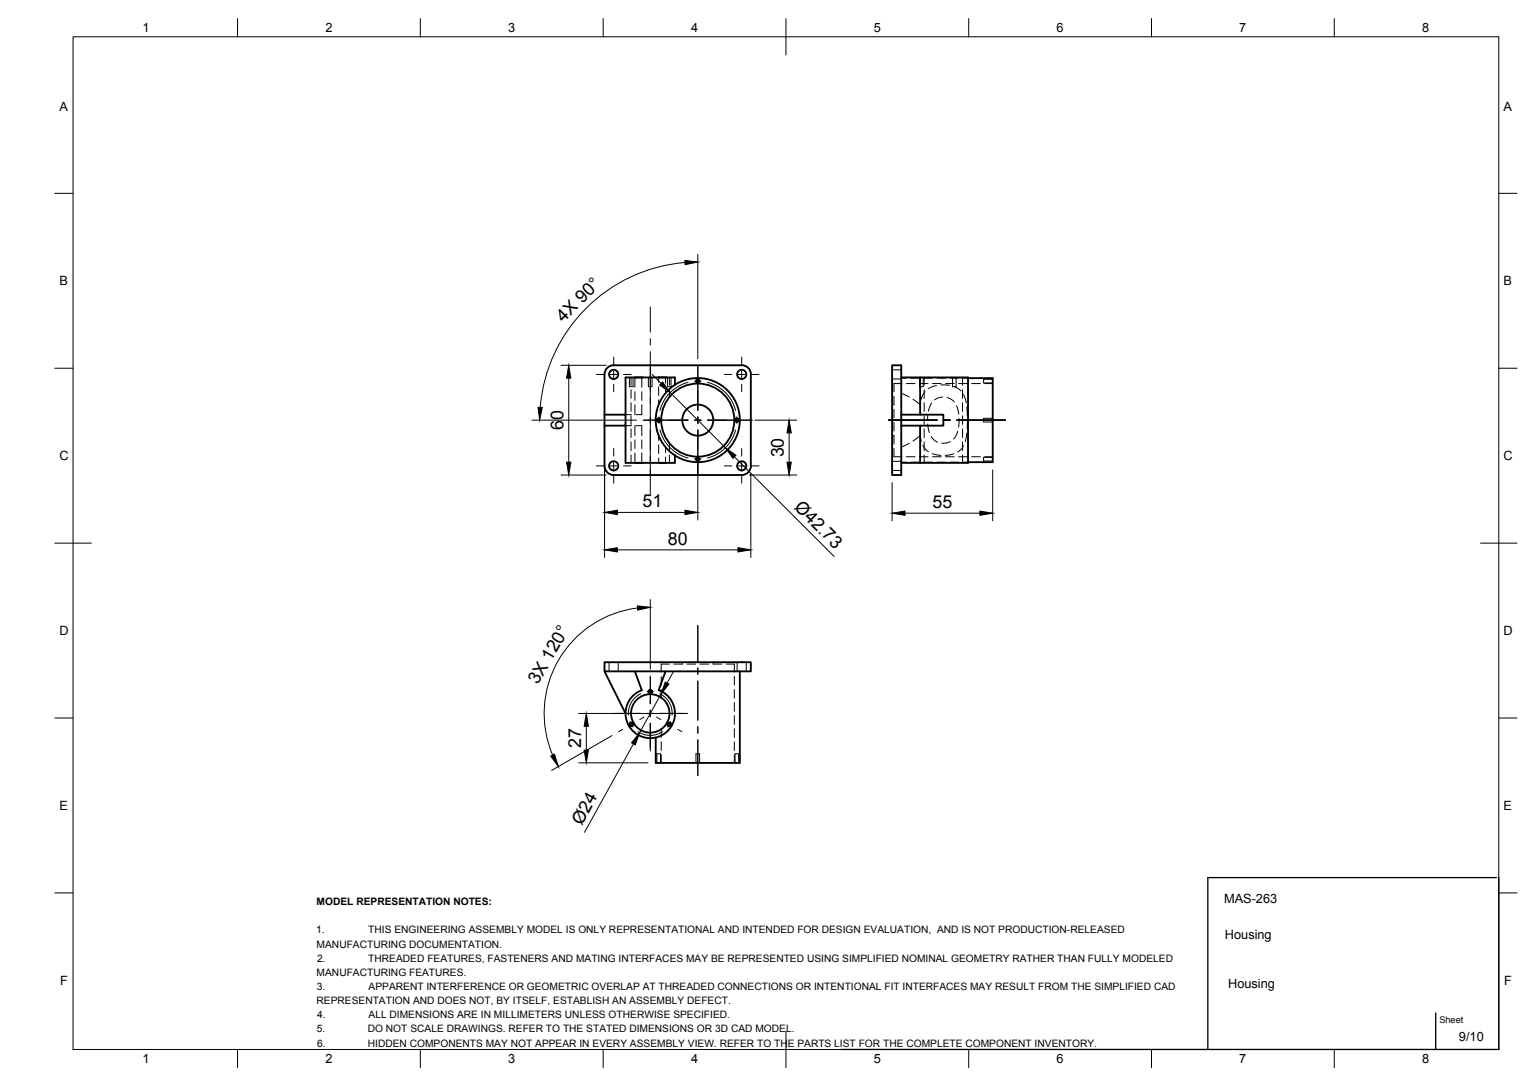
ISO-10303-21;
HEADER;
/* Generated by software containing ST-Developer
 * from STEP Tools, Inc. (www.steptools.com) 
 */

FILE_DESCRIPTION(
/* description */ (''),
/* implementation_level */ '2;1');

FILE_NAME(
/* name */ 'Housing.step',
/* time_stamp */ '2026-10-12T15:47:30-07:00',
/* author */ (''),
/* organization */ (''),
/* preprocessor_version */ 'ST-DEVELOPER v20.2',
/* originating_system */ 'Autodesk Translation Framework v15.15.0.0',
/* authorisation */ '');

FILE_SCHEMA (('AUTOMOTIVE_DESIGN { 1 0 10303 214 3 1 1 }'));
ENDSEC;

DATA;
#10=MECHANICAL_DESIGN_GEOMETRIC_PRESENTATION_REPRESENTATION('',(#87),#88483);
#69=SHAPE_REPRESENTATION_RELATIONSHIP('SRR','None',#88525,#78);
#78=ADVANCED_BREP_SHAPE_REPRESENTATION('',(#122),#88479);
#87=STYLED_ITEM('',(#88574),#122);
#122=MANIFOLD_SOLID_BREP('Body1',#12997);
#240=ELLIPSE('',#13948,67.247501203751,23.);
#241=ELLIPSE('',#13950,67.247501203751,23.);
#378=FACE_BOUND('',#1974,.T.);
#379=FACE_BOUND('',#1975,.T.);
#380=FACE_BOUND('',#1976,.T.);
#381=FACE_BOUND('',#1977,.T.);
#382=FACE_BOUND('',#1995,.T.);
#383=FACE_BOUND('',#1999,.T.);
#384=FACE_BOUND('',#2001,.T.);
#385=FACE_BOUND('',#2003,.T.);
#386=FACE_BOUND('',#2004,.T.);
#387=FACE_BOUND('',#2005,.T.);
#388=FACE_BOUND('',#2006,.T.);
#389=FACE_BOUND('',#2007,.T.);
#390=FACE_BOUND('',#2010,.T.);
#391=FACE_BOUND('',#2011,.T.);
#392=FACE_BOUND('',#2012,.T.);
#393=FACE_BOUND('',#2013,.T.);
#394=FACE_BOUND('',#2015,.T.);
#395=FACE_BOUND('',#2016,.T.);
#396=FACE_BOUND('',#2017,.T.);
#397=FACE_BOUND('',#2018,.T.);
#398=FACE_BOUND('',#2019,.T.);
#525=PLANE('',#13880);
#526=PLANE('',#13884);
#527=PLANE('',#13888);
#528=PLANE('',#13892);
#529=PLANE('',#13899);
#530=PLANE('',#13903);
#531=PLANE('',#13907);
#532=PLANE('',#13923);
#533=PLANE('',#13929);
#534=PLANE('',#13934);
#535=PLANE('',#13937);
#536=PLANE('',#13938);
#537=PLANE('',#13940);
#538=PLANE('',#13941);
#539=PLANE('',#13946);
#540=PLANE('',#13947);
#541=PLANE('',#13949);
#542=PLANE('',#13951);
#543=PLANE('',#13954);
#544=PLANE('',#13955);
#545=PLANE('',#13957);
#546=PLANE('',#13959);
#547=PLANE('',#13962);
#548=PLANE('',#13966);
#549=PLANE('',#13969);
#550=PLANE('',#13970);
#1256=FACE_OUTER_BOUND('',#1953,.T.);
#1257=FACE_OUTER_BOUND('',#1954,.T.);
#1258=FACE_OUTER_BOUND('',#1955,.T.);
#1259=FACE_OUTER_BOUND('',#1956,.T.);
#1260=FACE_OUTER_BOUND('',#1957,.T.);
#1261=FACE_OUTER_BOUND('',#1958,.T.);
#1262=FACE_OUTER_BOUND('',#1959,.T.);
#1263=FACE_OUTER_BOUND('',#1960,.T.);
#1264=FACE_OUTER_BOUND('',#1961,.T.);
#1265=FACE_OUTER_BOUND('',#1962,.T.);
#1266=FACE_OUTER_BOUND('',#1963,.T.);
#1267=FACE_OUTER_BOUND('',#1964,.T.);
#1268=FACE_OUTER_BOUND('',#1965,.T.);
#1269=FACE_OUTER_BOUND('',#1966,.T.);
#1270=FACE_OUTER_BOUND('',#1967,.T.);
#1271=FACE_OUTER_BOUND('',#1968,.T.);
#1272=FACE_OUTER_BOUND('',#1969,.T.);
#1273=FACE_OUTER_BOUND('',#1970,.T.);
#1274=FACE_OUTER_BOUND('',#1971,.T.);
#1275=FACE_OUTER_BOUND('',#1972,.T.);
#1276=FACE_OUTER_BOUND('',#1973,.T.);
#1277=FACE_OUTER_BOUND('',#1978,.T.);
#1278=FACE_OUTER_BOUND('',#1979,.T.);
#1279=FACE_OUTER_BOUND('',#1980,.T.);
#1280=FACE_OUTER_BOUND('',#1981,.T.);
#1281=FACE_OUTER_BOUND('',#1982,.T.);
#1282=FACE_OUTER_BOUND('',#1983,.T.);
#1283=FACE_OUTER_BOUND('',#1984,.T.);
#1284=FACE_OUTER_BOUND('',#1985,.T.);
#1285=FACE_OUTER_BOUND('',#1986,.T.);
#1286=FACE_OUTER_BOUND('',#1987,.T.);
#1287=FACE_OUTER_BOUND('',#1988,.T.);
#1288=FACE_OUTER_BOUND('',#1989,.T.);
#1289=FACE_OUTER_BOUND('',#1990,.T.);
#1290=FACE_OUTER_BOUND('',#1991,.T.);
#1291=FACE_OUTER_BOUND('',#1992,.T.);
#1292=FACE_OUTER_BOUND('',#1993,.T.);
#1293=FACE_OUTER_BOUND('',#1994,.T.);
#1294=FACE_OUTER_BOUND('',#1996,.T.);
#1295=FACE_OUTER_BOUND('',#1997,.T.);
#1296=FACE_OUTER_BOUND('',#1998,.T.);
#1297=FACE_OUTER_BOUND('',#2000,.T.);
#1298=FACE_OUTER_BOUND('',#2002,.T.);
#1299=FACE_OUTER_BOUND('',#2008,.T.);
#1300=FACE_OUTER_BOUND('',#2009,.T.);
#1301=FACE_OUTER_BOUND('',#2014,.T.);
#1953=EDGE_LOOP('',(#11238,#11239,#11240,#11241));
#1954=EDGE_LOOP('',(#11242));
#1955=EDGE_LOOP('',(#11243,#11244,#11245,#11246));
#1956=EDGE_LOOP('',(#11247));
#1957=EDGE_LOOP('',(#11248,#11249,#11250,#11251));
#1958=EDGE_LOOP('',(#11252));
#1959=EDGE_LOOP('',(#11253,#11254,#11255,#11256));
#1960=EDGE_LOOP('',(#11257));
#1961=EDGE_LOOP('',(#11258,#11259,#11260,#11261));
#1962=EDGE_LOOP('',(#11262,#11263,#11264,#11265));
#1963=EDGE_LOOP('',(#11266));
#1964=EDGE_LOOP('',(#11267,#11268,#11269,#11270));
#1965=EDGE_LOOP('',(#11271));
#1966=EDGE_LOOP('',(#11272,#11273,#11274,#11275));
#1967=EDGE_LOOP('',(#11276));
#1968=EDGE_LOOP('',(#11277,#11278,#11279,#11280));
#1969=EDGE_LOOP('',(#11281,#11282,#11283,#11284));
#1970=EDGE_LOOP('',(#11285,#11286,#11287,#11288));
#1971=EDGE_LOOP('',(#11289,#11290,#11291,#11292));
#1972=EDGE_LOOP('',(#11293,#11294,#11295,#11296));
#1973=EDGE_LOOP('',(#11297,#11298,#11299,#11300,#11301,#11302,#11303,#11304,
#11305,#11306,#11307,#11308,#11309,#11310,#11311,#11312,#11313,#11314,#11315));
#1974=EDGE_LOOP('',(#11316));
#1975=EDGE_LOOP('',(#11317));
#1976=EDGE_LOOP('',(#11318));
#1977=EDGE_LOOP('',(#11319));
#1978=EDGE_LOOP('',(#11320,#11321,#11322,#11323));
#1979=EDGE_LOOP('',(#11324,#11325,#11326,#11327));
#1980=EDGE_LOOP('',(#11328,#11329,#11330,#11331));
#1981=EDGE_LOOP('',(#11332,#11333,#11334,#11335,#11336,#11337));
#1982=EDGE_LOOP('',(#11338,#11339,#11340,#11341));
#1983=EDGE_LOOP('',(#11342,#11343,#11344,#11345));
#1984=EDGE_LOOP('',(#11346,#11347,#11348,#11349));
#1985=EDGE_LOOP('',(#11350,#11351,#11352,#11353));
#1986=EDGE_LOOP('',(#11354,#11355,#11356,#11357));
#1987=EDGE_LOOP('',(#11358,#11359,#11360,#11361,#11362,#11363,#11364,#11365,
#11366,#11367));
#1988=EDGE_LOOP('',(#11368,#11369,#11370,#11371));
#1989=EDGE_LOOP('',(#11372,#11373,#11374,#11375));
#1990=EDGE_LOOP('',(#11376,#11377,#11378,#11379));
#1991=EDGE_LOOP('',(#11380,#11381,#11382,#11383,#11384));
#1992=EDGE_LOOP('',(#11385,#11386,#11387,#11388));
#1993=EDGE_LOOP('',(#11389,#11390,#11391,#11392));
#1994=EDGE_LOOP('',(#11393,#11394,#11395));
#1995=EDGE_LOOP('',(#11396));
#1996=EDGE_LOOP('',(#11397,#11398,#11399,#11400));
#1997=EDGE_LOOP('',(#11401,#11402,#11403,#11404,#11405,#11406,#11407,#11408,
#11409));
#1998=EDGE_LOOP('',(#11410));
#1999=EDGE_LOOP('',(#11411));
#2000=EDGE_LOOP('',(#11412,#11413,#11414,#11415));
#2001=EDGE_LOOP('',(#11416,#11417,#11418));
#2002=EDGE_LOOP('',(#11419));
#2003=EDGE_LOOP('',(#11420));
#2004=EDGE_LOOP('',(#11421));
#2005=EDGE_LOOP('',(#11422));
#2006=EDGE_LOOP('',(#11423));
#2007=EDGE_LOOP('',(#11424));
#2008=EDGE_LOOP('',(#11425,#11426,#11427,#11428,#11429,#11430,#11431,#11432));
#2009=EDGE_LOOP('',(#11433,#11434));
#2010=EDGE_LOOP('',(#11435));
#2011=EDGE_LOOP('',(#11436));
#2012=EDGE_LOOP('',(#11437));
#2013=EDGE_LOOP('',(#11438));
#2014=EDGE_LOOP('',(#11439,#11440,#11441,#11442,#11443,#11444,#11445,#11446));
#2015=EDGE_LOOP('',(#11447));
#2016=EDGE_LOOP('',(#11448));
#2017=EDGE_LOOP('',(#11449));
#2018=EDGE_LOOP('',(#11450));
#2019=EDGE_LOOP('',(#11451));
#2640=CIRCLE('',#13878,1.);
#2641=CIRCLE('',#13879,1.);
#2642=CIRCLE('',#13882,1.);
#2643=CIRCLE('',#13883,1.);
#2644=CIRCLE('',#13886,1.);
#2645=CIRCLE('',#13887,1.);
#2646=CIRCLE('',#13890,1.);
#2647=CIRCLE('',#13891,1.);
#2648=CIRCLE('',#13894,8.5);
#2649=CIRCLE('',#13895,8.5);
#2650=CIRCLE('',#13897,1.);
#2651=CIRCLE('',#13898,1.);
#2652=CIRCLE('',#13901,1.);
#2653=CIRCLE('',#13902,1.);
#2654=CIRCLE('',#13905,1.);
#2655=CIRCLE('',#13906,1.);
#2656=CIRCLE('',#13909,2.5);
#2657=CIRCLE('',#13910,2.5);
#2658=CIRCLE('',#13912,2.5);
#2659=CIRCLE('',#13913,2.5);
#2660=CIRCLE('',#13915,2.5);
#2661=CIRCLE('',#13916,2.5);
#2662=CIRCLE('',#13918,2.5);
#2663=CIRCLE('',#13919,2.5);
#2664=CIRCLE('',#13921,5.);
#2665=CIRCLE('',#13922,5.);
#2666=CIRCLE('',#13924,5.);
#2667=CIRCLE('',#13925,5.);
#2668=CIRCLE('',#13926,23.);
#2669=CIRCLE('',#13927,23.);
#2670=CIRCLE('',#13928,5.);
#2671=CIRCLE('',#13931,5.);
#2672=CIRCLE('',#13933,5.);
#2673=CIRCLE('',#13936,5.);
#2674=CIRCLE('',#13939,13.5);
#2675=CIRCLE('',#13942,13.5);
#2676=CIRCLE('',#13944,13.5);
#2677=CIRCLE('',#13945,13.5);
#2678=CIRCLE('',#13952,13.5);
#2679=CIRCLE('',#13953,13.5);
#2680=CIRCLE('',#13956,13.5);
#2681=CIRCLE('',#13958,10.5);
#2682=CIRCLE('',#13961,10.5);
#2683=CIRCLE('',#13963,20.);
#2684=CIRCLE('',#13965,20.);
#2685=CIRCLE('',#13967,23.);
#3627=B_SPLINE_CURVE_WITH_KNOTS('',3,(#87301,#87302,#87303,#87304,#87305,
#87306,#87307,#87308,#87309,#87310,#87311,#87312,#87313,#87314,#87315,#87316,
#87317,#87318,#87319,#87320,#87321,#87322,#87323,#87324,#87325,#87326,#87327,
#87328,#87329,#87330,#87331,#87332,#87333,#87334,#87335,#87336,#87337,#87338,
#87339,#87340,#87341,#87342,#87343,#87344,#87345,#87346,#87347,#87348,#87349,
#87350,#87351,#87352,#87353,#87354,#87355,#87356,#87357,#87358,#87359),
 .UNSPECIFIED.,.F.,.F.,(4,2,2,2,2,2,2,2,2,2,2,2,2,2,3,2,2,2,2,2,2,2,2,2,
2,2,2,2,4),(-4.85232699494737,-4.58025935130269,-4.21243389208218,-3.93854775205376,
-3.66466161202534,-3.25326473825372,-2.84186786448211,-2.43047099071049,
-2.01907411693888,-1.74518797691046,-1.47130183688203,-1.10347637766153,
-0.735650918441017,-0.367825459220508,0.,0.367825459220509,0.735650918441017,
1.10347637766153,1.47130183688203,1.74518797691046,2.01907411693888,2.43047099071049,
2.84186786448211,3.25326473825372,3.66466161202534,3.93854775205376,4.21243389208218,
4.58025935130269,4.85232699494738),.UNSPECIFIED.);
#3628=B_SPLINE_CURVE_WITH_KNOTS('',3,(#87390,#87391,#87392,#87393,#87394,
#87395,#87396,#87397,#87398,#87399,#87400,#87401,#87402,#87403),
 .UNSPECIFIED.,.F.,.F.,(4,2,2,2,2,2,4),(8.79034115467969,9.02147795200396,
9.25261474932822,9.57656340840008,9.90051206747193,10.2244607265438,10.5484093856156),
 .UNSPECIFIED.);
#3629=B_SPLINE_CURVE_WITH_KNOTS('',3,(#87405,#87406,#87407,#87408,#87409,
#87410,#87411,#87412,#87413,#87414,#87415,#87416,#87417,#87418),
 .UNSPECIFIED.,.F.,.F.,(4,2,2,2,2,2,4),(3.51613646187188,3.84008512094373,
4.16403378001558,4.48798243908744,4.81193109815929,5.04306789548355,5.27420469280782),
 .UNSPECIFIED.);
#3630=B_SPLINE_CURVE_WITH_KNOTS('',3,(#87422,#87423,#87424,#87425,#87426,
#87427,#87428,#87429,#87430,#87431,#87432,#87433,#87434,#87435,#87436,#87437,
#87438,#87439,#87440,#87441,#87442,#87443,#87444,#87445,#87446,#87447,#87448),
 .UNSPECIFIED.,.F.,.F.,(4,2,2,2,2,2,3,2,2,2,2,2,4),(5.27420469280782,5.50534149013208,
5.73647828745635,6.0604269465282,6.38437560560005,6.7083242646719,7.03227292374376,
7.35622158281561,7.68017024188746,8.00411890095931,8.32806756003117,8.55920435735543,
8.79034115467969),.UNSPECIFIED.);
#4034=LINE('',#87134,#4504);
#4035=LINE('',#87141,#4505);
#4036=LINE('',#87148,#4506);
#4037=LINE('',#87155,#4507);
#4038=LINE('',#87162,#4508);
#4039=LINE('',#87168,#4509);
#4040=LINE('',#87175,#4510);
#4041=LINE('',#87182,#4511);
#4042=LINE('',#87189,#4512);
#4043=LINE('',#87195,#4513);
#4044=LINE('',#87201,#4514);
#4045=LINE('',#87207,#4515);
#4046=LINE('',#87214,#4516);
#4047=LINE('',#87217,#4517);
#4048=LINE('',#87220,#4518);
#4049=LINE('',#87224,#4519);
#4050=LINE('',#87228,#4520);
#4051=LINE('',#87230,#4521);
#4052=LINE('',#87232,#4522);
#4053=LINE('',#87234,#4523);
#4054=LINE('',#87236,#4524);
#4055=LINE('',#87242,#4525);
#4056=LINE('',#87244,#4526);
#4057=LINE('',#87246,#4527);
#4058=LINE('',#87248,#4528);
#4059=LINE('',#87250,#4529);
#4060=LINE('',#87253,#4530);
#4061=LINE('',#87256,#4531);
#4062=LINE('',#87257,#4532);
#4063=LINE('',#87261,#4533);
#4064=LINE('',#87266,#4534);
#4065=LINE('',#87267,#4535);
#4066=LINE('',#87269,#4536);
#4067=LINE('',#87271,#4537);
#4068=LINE('',#87272,#4538);
#4069=LINE('',#87276,#4539);
#4070=LINE('',#87278,#4540);
#4071=LINE('',#87281,#4541);
#4072=LINE('',#87284,#4542);
#4073=LINE('',#87287,#4543);
#4074=LINE('',#87288,#4544);
#4075=LINE('',#87292,#4545);
#4076=LINE('',#87295,#4546);
#4077=LINE('',#87299,#4547);
#4078=LINE('',#87361,#4548);
#4079=LINE('',#87364,#4549);
#4080=LINE('',#87366,#4550);
#4081=LINE('',#87369,#4551);
#4082=LINE('',#87371,#4552);
#4083=LINE('',#87378,#4553);
#4084=LINE('',#87385,#4554);
#4085=LINE('',#87388,#4555);
#4086=LINE('',#87420,#4556);
#4087=LINE('',#87454,#4557);
#4088=LINE('',#87460,#4558);
#4504=VECTOR('',#16242,1.);
#4505=VECTOR('',#16251,1.);
#4506=VECTOR('',#16260,1.);
#4507=VECTOR('',#16269,1.);
#4508=VECTOR('',#16278,8.5);
#4509=VECTOR('',#16285,1.);
#4510=VECTOR('',#16294,1.);
#4511=VECTOR('',#16303,1.);
#4512=VECTOR('',#16312,2.5);
#4513=VECTOR('',#16319,2.5);
#4514=VECTOR('',#16326,2.5);
#4515=VECTOR('',#16333,2.5);
#4516=VECTOR('',#16340,10.);
#4517=VECTOR('',#16343,10.);
#4518=VECTOR('',#16346,10.);
#4519=VECTOR('',#16349,10.);
#4520=VECTOR('',#16352,10.);
#4521=VECTOR('',#16353,10.);
#4522=VECTOR('',#16354,10.);
#4523=VECTOR('',#16355,10.);
#4524=VECTOR('',#16356,10.);
#4525=VECTOR('',#16361,10.);
#4526=VECTOR('',#16362,10.);
#4527=VECTOR('',#16363,10.);
#4528=VECTOR('',#16364,10.);
#4529=VECTOR('',#16365,10.);
#4530=VECTOR('',#16368,10.);
#4531=VECTOR('',#16371,10.);
#4532=VECTOR('',#16372,10.);
#4533=VECTOR('',#16377,10.);
#4534=VECTOR('',#16382,10.);
#4535=VECTOR('',#16383,10.);
#4536=VECTOR('',#16386,10.);
#4537=VECTOR('',#16387,10.);
#4538=VECTOR('',#16388,10.);
#4539=VECTOR('',#16393,10.);
#4540=VECTOR('',#16396,10.);
#4541=VECTOR('',#16399,10.);
#4542=VECTOR('',#16402,10.);
#4543=VECTOR('',#16405,10.);
#4544=VECTOR('',#16406,10.);
#4545=VECTOR('',#16411,10.);
#4546=VECTOR('',#16414,10.);
#4547=VECTOR('',#16417,10.);
#4548=VECTOR('',#16418,10.);
#4549=VECTOR('',#16421,10.);
#4550=VECTOR('',#16424,10.);
#4551=VECTOR('',#16429,10.);
#4552=VECTOR('',#16432,10.);
#4553=VECTOR('',#16443,10.);
#4554=VECTOR('',#16454,10.);
#4555=VECTOR('',#16457,10.5);
#4556=VECTOR('',#16458,10.5);
#4557=VECTOR('',#16467,20.);
#4558=VECTOR('',#16476,23.);
#5751=VERTEX_POINT('',#87131);
#5752=VERTEX_POINT('',#87133);
#5753=VERTEX_POINT('',#87138);
#5754=VERTEX_POINT('',#87140);
#5755=VERTEX_POINT('',#87145);
#5756=VERTEX_POINT('',#87147);
#5757=VERTEX_POINT('',#87152);
#5758=VERTEX_POINT('',#87154);
#5759=VERTEX_POINT('',#87159);
#5760=VERTEX_POINT('',#87161);
#5761=VERTEX_POINT('',#87165);
#5762=VERTEX_POINT('',#87167);
#5763=VERTEX_POINT('',#87172);
#5764=VERTEX_POINT('',#87174);
#5765=VERTEX_POINT('',#87179);
#5766=VERTEX_POINT('',#87181);
#5767=VERTEX_POINT('',#87186);
#5768=VERTEX_POINT('',#87188);
#5769=VERTEX_POINT('',#87192);
#5770=VERTEX_POINT('',#87194);
#5771=VERTEX_POINT('',#87198);
#5772=VERTEX_POINT('',#87200);
#5773=VERTEX_POINT('',#87204);
#5774=VERTEX_POINT('',#87206);
#5775=VERTEX_POINT('',#87210);
#5776=VERTEX_POINT('',#87211);
#5777=VERTEX_POINT('',#87213);
#5778=VERTEX_POINT('',#87215);
#5779=VERTEX_POINT('',#87219);
#5780=VERTEX_POINT('',#87221);
#5781=VERTEX_POINT('',#87223);
#5782=VERTEX_POINT('',#87225);
#5783=VERTEX_POINT('',#87227);
#5784=VERTEX_POINT('',#87229);
#5785=VERTEX_POINT('',#87231);
#5786=VERTEX_POINT('',#87233);
#5787=VERTEX_POINT('',#87235);
#5788=VERTEX_POINT('',#87237);
#5789=VERTEX_POINT('',#87239);
#5790=VERTEX_POINT('',#87241);
#5791=VERTEX_POINT('',#87243);
#5792=VERTEX_POINT('',#87245);
#5793=VERTEX_POINT('',#87247);
#5794=VERTEX_POINT('',#87249);
#5795=VERTEX_POINT('',#87251);
#5796=VERTEX_POINT('',#87255);
#5797=VERTEX_POINT('',#87259);
#5798=VERTEX_POINT('',#87263);
#5799=VERTEX_POINT('',#87264);
#5800=VERTEX_POINT('',#87270);
#5801=VERTEX_POINT('',#87274);
#5802=VERTEX_POINT('',#87280);
#5803=VERTEX_POINT('',#87282);
#5804=VERTEX_POINT('',#87286);
#5805=VERTEX_POINT('',#87290);
#5806=VERTEX_POINT('',#87294);
#5807=VERTEX_POINT('',#87296);
#5808=VERTEX_POINT('',#87298);
#5809=VERTEX_POINT('',#87300);
#5810=VERTEX_POINT('',#87360);
#5811=VERTEX_POINT('',#87362);
#5812=VERTEX_POINT('',#87374);
#5813=VERTEX_POINT('',#87382);
#5814=VERTEX_POINT('',#87387);
#5815=VERTEX_POINT('',#87389);
#5816=VERTEX_POINT('',#87404);
#5817=VERTEX_POINT('',#87419);
#5818=VERTEX_POINT('',#87450);
#5819=VERTEX_POINT('',#87453);
#5820=VERTEX_POINT('',#87457);
#7631=EDGE_CURVE('',#5751,#5751,#2640,.T.);
#7632=EDGE_CURVE('',#5751,#5752,#4034,.T.);
#7633=EDGE_CURVE('',#5752,#5752,#2641,.T.);
#7634=EDGE_CURVE('',#5753,#5753,#2642,.T.);
#7635=EDGE_CURVE('',#5753,#5754,#4035,.T.);
#7636=EDGE_CURVE('',#5754,#5754,#2643,.T.);
#7637=EDGE_CURVE('',#5755,#5755,#2644,.T.);
#7638=EDGE_CURVE('',#5755,#5756,#4036,.T.);
#7639=EDGE_CURVE('',#5756,#5756,#2645,.T.);
#7640=EDGE_CURVE('',#5757,#5757,#2646,.T.);
#7641=EDGE_CURVE('',#5757,#5758,#4037,.T.);
#7642=EDGE_CURVE('',#5758,#5758,#2647,.T.);
#7643=EDGE_CURVE('',#5759,#5759,#2648,.T.);
#7644=EDGE_CURVE('',#5759,#5760,#4038,.T.);
#7645=EDGE_CURVE('',#5760,#5760,#2649,.T.);
#7646=EDGE_CURVE('',#5761,#5761,#2650,.T.);
#7647=EDGE_CURVE('',#5761,#5762,#4039,.T.);
#7648=EDGE_CURVE('',#5762,#5762,#2651,.T.);
#7649=EDGE_CURVE('',#5763,#5763,#2652,.T.);
#7650=EDGE_CURVE('',#5763,#5764,#4040,.T.);
#7651=EDGE_CURVE('',#5764,#5764,#2653,.T.);
#7652=EDGE_CURVE('',#5765,#5765,#2654,.T.);
#7653=EDGE_CURVE('',#5765,#5766,#4041,.T.);
#7654=EDGE_CURVE('',#5766,#5766,#2655,.T.);
#7655=EDGE_CURVE('',#5767,#5767,#2656,.T.);
#7656=EDGE_CURVE('',#5767,#5768,#4042,.T.);
#7657=EDGE_CURVE('',#5768,#5768,#2657,.T.);
#7658=EDGE_CURVE('',#5769,#5769,#2658,.T.);
#7659=EDGE_CURVE('',#5769,#5770,#4043,.T.);
#7660=EDGE_CURVE('',#5770,#5770,#2659,.T.);
#7661=EDGE_CURVE('',#5771,#5771,#2660,.T.);
#7662=EDGE_CURVE('',#5771,#5772,#4044,.T.);
#7663=EDGE_CURVE('',#5772,#5772,#2661,.T.);
#7664=EDGE_CURVE('',#5773,#5773,#2662,.T.);
#7665=EDGE_CURVE('',#5773,#5774,#4045,.T.);
#7666=EDGE_CURVE('',#5774,#5774,#2663,.T.);
#7667=EDGE_CURVE('',#5775,#5776,#2664,.T.);
#7668=EDGE_CURVE('',#5776,#5777,#4046,.T.);
#7669=EDGE_CURVE('',#5777,#5778,#2665,.T.);
#7670=EDGE_CURVE('',#5778,#5775,#4047,.T.);
#7671=EDGE_CURVE('',#5777,#5779,#4048,.T.);
#7672=EDGE_CURVE('',#5780,#5779,#2666,.T.);
#7673=EDGE_CURVE('',#5780,#5781,#4049,.T.);
#7674=EDGE_CURVE('',#5782,#5781,#2667,.T.);
#7675=EDGE_CURVE('',#5782,#5783,#4050,.T.);
#7676=EDGE_CURVE('',#5783,#5784,#4051,.T.);
#7677=EDGE_CURVE('',#5784,#5785,#4052,.T.);
#7678=EDGE_CURVE('',#5785,#5786,#4053,.T.);
#7679=EDGE_CURVE('',#5786,#5787,#4054,.T.);
#7680=EDGE_CURVE('',#5787,#5788,#2668,.T.);
#7681=EDGE_CURVE('',#5788,#5789,#2669,.T.);
#7682=EDGE_CURVE('',#5789,#5790,#4055,.T.);
#7683=EDGE_CURVE('',#5790,#5791,#4056,.T.);
#7684=EDGE_CURVE('',#5791,#5792,#4057,.T.);
#7685=EDGE_CURVE('',#5792,#5793,#4058,.T.);
#7686=EDGE_CURVE('',#5793,#5794,#4059,.T.);
#7687=EDGE_CURVE('',#5795,#5794,#2670,.T.);
#7688=EDGE_CURVE('',#5778,#5795,#4060,.T.);
#7689=EDGE_CURVE('',#5796,#5776,#4061,.T.);
#7690=EDGE_CURVE('',#5779,#5796,#4062,.T.);
#7691=EDGE_CURVE('',#5796,#5797,#2671,.T.);
#7692=EDGE_CURVE('',#5797,#5780,#4063,.T.);
#7693=EDGE_CURVE('',#5798,#5799,#2672,.T.);
#7694=EDGE_CURVE('',#5799,#5795,#4064,.T.);
#7695=EDGE_CURVE('',#5794,#5798,#4065,.T.);
#7696=EDGE_CURVE('',#5783,#5793,#4066,.T.);
#7697=EDGE_CURVE('',#5800,#5782,#4067,.T.);
#7698=EDGE_CURVE('',#5798,#5800,#4068,.T.);
#7699=EDGE_CURVE('',#5801,#5800,#2673,.T.);
#7700=EDGE_CURVE('',#5781,#5801,#4069,.T.);
#7701=EDGE_CURVE('',#5801,#5797,#4070,.T.);
#7702=EDGE_CURVE('',#5802,#5792,#4071,.T.);
#7703=EDGE_CURVE('',#5803,#5802,#2674,.T.);
#7704=EDGE_CURVE('',#5803,#5793,#4072,.T.);
#7705=EDGE_CURVE('',#5804,#5803,#4073,.T.);
#7706=EDGE_CURVE('',#5783,#5804,#4074,.T.);
#7707=EDGE_CURVE('',#5805,#5804,#2675,.T.);
#7708=EDGE_CURVE('',#5784,#5805,#4075,.T.);
#7709=EDGE_CURVE('',#5802,#5806,#4076,.T.);
#7710=EDGE_CURVE('',#5807,#5806,#2676,.T.);
#7711=EDGE_CURVE('',#5807,#5808,#4077,.T.);
#7712=EDGE_CURVE('',#5809,#5808,#3627,.F.);
#7713=EDGE_CURVE('',#5809,#5810,#4078,.T.);
#7714=EDGE_CURVE('',#5810,#5811,#2677,.T.);
#7715=EDGE_CURVE('',#5811,#5805,#4079,.T.);
#7716=EDGE_CURVE('',#5806,#5791,#4080,.T.);
#7717=EDGE_CURVE('',#5787,#5809,#240,.F.);
#7718=EDGE_CURVE('',#5810,#5786,#4081,.T.);
#7719=EDGE_CURVE('',#5790,#5807,#4082,.T.);
#7720=EDGE_CURVE('',#5808,#5789,#241,.F.);
#7721=EDGE_CURVE('',#5812,#5806,#2678,.T.);
#7722=EDGE_CURVE('',#5812,#5807,#2679,.T.);
#7723=EDGE_CURVE('',#5785,#5811,#4083,.T.);
#7724=EDGE_CURVE('',#5811,#5810,#2680,.T.);
#7725=EDGE_CURVE('',#5813,#5813,#2681,.T.);
#7726=EDGE_CURVE('',#5799,#5775,#4084,.T.);
#7727=EDGE_CURVE('',#5813,#5814,#4085,.T.);
#7728=EDGE_CURVE('',#5815,#5814,#3628,.F.);
#7729=EDGE_CURVE('',#5816,#5815,#3629,.F.);
#7730=EDGE_CURVE('',#5816,#5817,#4086,.T.);
#7731=EDGE_CURVE('',#5817,#5817,#2682,.T.);
#7732=EDGE_CURVE('',#5814,#5816,#3630,.F.);
#7733=EDGE_CURVE('',#5818,#5818,#2683,.F.);
#7734=EDGE_CURVE('',#5818,#5819,#4087,.T.);
#7735=EDGE_CURVE('',#5819,#5819,#2684,.T.);
#7736=EDGE_CURVE('',#5820,#5820,#2685,.T.);
#7737=EDGE_CURVE('',#5820,#5788,#4088,.T.);
#11238=ORIENTED_EDGE('',*,*,#7631,.F.);
#11239=ORIENTED_EDGE('',*,*,#7632,.T.);
#11240=ORIENTED_EDGE('',*,*,#7633,.T.);
#11241=ORIENTED_EDGE('',*,*,#7632,.F.);
#11242=ORIENTED_EDGE('',*,*,#7633,.F.);
#11243=ORIENTED_EDGE('',*,*,#7634,.F.);
#11244=ORIENTED_EDGE('',*,*,#7635,.T.);
#11245=ORIENTED_EDGE('',*,*,#7636,.T.);
#11246=ORIENTED_EDGE('',*,*,#7635,.F.);
#11247=ORIENTED_EDGE('',*,*,#7636,.F.);
#11248=ORIENTED_EDGE('',*,*,#7637,.F.);
#11249=ORIENTED_EDGE('',*,*,#7638,.T.);
#11250=ORIENTED_EDGE('',*,*,#7639,.T.);
#11251=ORIENTED_EDGE('',*,*,#7638,.F.);
#11252=ORIENTED_EDGE('',*,*,#7639,.F.);
#11253=ORIENTED_EDGE('',*,*,#7640,.F.);
#11254=ORIENTED_EDGE('',*,*,#7641,.T.);
#11255=ORIENTED_EDGE('',*,*,#7642,.T.);
#11256=ORIENTED_EDGE('',*,*,#7641,.F.);
#11257=ORIENTED_EDGE('',*,*,#7642,.F.);
#11258=ORIENTED_EDGE('',*,*,#7643,.F.);
#11259=ORIENTED_EDGE('',*,*,#7644,.T.);
#11260=ORIENTED_EDGE('',*,*,#7645,.F.);
#11261=ORIENTED_EDGE('',*,*,#7644,.F.);
#11262=ORIENTED_EDGE('',*,*,#7646,.F.);
#11263=ORIENTED_EDGE('',*,*,#7647,.T.);
#11264=ORIENTED_EDGE('',*,*,#7648,.T.);
#11265=ORIENTED_EDGE('',*,*,#7647,.F.);
#11266=ORIENTED_EDGE('',*,*,#7648,.F.);
#11267=ORIENTED_EDGE('',*,*,#7649,.F.);
#11268=ORIENTED_EDGE('',*,*,#7650,.T.);
#11269=ORIENTED_EDGE('',*,*,#7651,.T.);
#11270=ORIENTED_EDGE('',*,*,#7650,.F.);
#11271=ORIENTED_EDGE('',*,*,#7651,.F.);
#11272=ORIENTED_EDGE('',*,*,#7652,.F.);
#11273=ORIENTED_EDGE('',*,*,#7653,.T.);
#11274=ORIENTED_EDGE('',*,*,#7654,.T.);
#11275=ORIENTED_EDGE('',*,*,#7653,.F.);
#11276=ORIENTED_EDGE('',*,*,#7654,.F.);
#11277=ORIENTED_EDGE('',*,*,#7655,.F.);
#11278=ORIENTED_EDGE('',*,*,#7656,.T.);
#11279=ORIENTED_EDGE('',*,*,#7657,.F.);
#11280=ORIENTED_EDGE('',*,*,#7656,.F.);
#11281=ORIENTED_EDGE('',*,*,#7658,.F.);
#11282=ORIENTED_EDGE('',*,*,#7659,.T.);
#11283=ORIENTED_EDGE('',*,*,#7660,.F.);
#11284=ORIENTED_EDGE('',*,*,#7659,.F.);
#11285=ORIENTED_EDGE('',*,*,#7661,.F.);
#11286=ORIENTED_EDGE('',*,*,#7662,.T.);
#11287=ORIENTED_EDGE('',*,*,#7663,.F.);
#11288=ORIENTED_EDGE('',*,*,#7662,.F.);
#11289=ORIENTED_EDGE('',*,*,#7664,.F.);
#11290=ORIENTED_EDGE('',*,*,#7665,.T.);
#11291=ORIENTED_EDGE('',*,*,#7666,.F.);
#11292=ORIENTED_EDGE('',*,*,#7665,.F.);
#11293=ORIENTED_EDGE('',*,*,#7667,.T.);
#11294=ORIENTED_EDGE('',*,*,#7668,.T.);
#11295=ORIENTED_EDGE('',*,*,#7669,.T.);
#11296=ORIENTED_EDGE('',*,*,#7670,.T.);
#11297=ORIENTED_EDGE('',*,*,#7669,.F.);
#11298=ORIENTED_EDGE('',*,*,#7671,.T.);
#11299=ORIENTED_EDGE('',*,*,#7672,.F.);
#11300=ORIENTED_EDGE('',*,*,#7673,.T.);
#11301=ORIENTED_EDGE('',*,*,#7674,.F.);
#11302=ORIENTED_EDGE('',*,*,#7675,.T.);
#11303=ORIENTED_EDGE('',*,*,#7676,.T.);
#11304=ORIENTED_EDGE('',*,*,#7677,.T.);
#11305=ORIENTED_EDGE('',*,*,#7678,.T.);
#11306=ORIENTED_EDGE('',*,*,#7679,.T.);
#11307=ORIENTED_EDGE('',*,*,#7680,.T.);
#11308=ORIENTED_EDGE('',*,*,#7681,.T.);
#11309=ORIENTED_EDGE('',*,*,#7682,.T.);
#11310=ORIENTED_EDGE('',*,*,#7683,.T.);
#11311=ORIENTED_EDGE('',*,*,#7684,.T.);
#11312=ORIENTED_EDGE('',*,*,#7685,.T.);
#11313=ORIENTED_EDGE('',*,*,#7686,.T.);
#11314=ORIENTED_EDGE('',*,*,#7687,.F.);
#11315=ORIENTED_EDGE('',*,*,#7688,.F.);
#11316=ORIENTED_EDGE('',*,*,#7655,.T.);
#11317=ORIENTED_EDGE('',*,*,#7658,.T.);
#11318=ORIENTED_EDGE('',*,*,#7661,.T.);
#11319=ORIENTED_EDGE('',*,*,#7664,.T.);
#11320=ORIENTED_EDGE('',*,*,#7668,.F.);
#11321=ORIENTED_EDGE('',*,*,#7689,.F.);
#11322=ORIENTED_EDGE('',*,*,#7690,.F.);
#11323=ORIENTED_EDGE('',*,*,#7671,.F.);
#11324=ORIENTED_EDGE('',*,*,#7691,.T.);
#11325=ORIENTED_EDGE('',*,*,#7692,.T.);
#11326=ORIENTED_EDGE('',*,*,#7672,.T.);
#11327=ORIENTED_EDGE('',*,*,#7690,.T.);
#11328=ORIENTED_EDGE('',*,*,#7693,.T.);
#11329=ORIENTED_EDGE('',*,*,#7694,.T.);
#11330=ORIENTED_EDGE('',*,*,#7687,.T.);
#11331=ORIENTED_EDGE('',*,*,#7695,.T.);
#11332=ORIENTED_EDGE('',*,*,#7695,.F.);
#11333=ORIENTED_EDGE('',*,*,#7686,.F.);
#11334=ORIENTED_EDGE('',*,*,#7696,.F.);
#11335=ORIENTED_EDGE('',*,*,#7675,.F.);
#11336=ORIENTED_EDGE('',*,*,#7697,.F.);
#11337=ORIENTED_EDGE('',*,*,#7698,.F.);
#11338=ORIENTED_EDGE('',*,*,#7699,.T.);
#11339=ORIENTED_EDGE('',*,*,#7697,.T.);
#11340=ORIENTED_EDGE('',*,*,#7674,.T.);
#11341=ORIENTED_EDGE('',*,*,#7700,.T.);
#11342=ORIENTED_EDGE('',*,*,#7692,.F.);
#11343=ORIENTED_EDGE('',*,*,#7701,.F.);
#11344=ORIENTED_EDGE('',*,*,#7700,.F.);
#11345=ORIENTED_EDGE('',*,*,#7673,.F.);
#11346=ORIENTED_EDGE('',*,*,#7685,.F.);
#11347=ORIENTED_EDGE('',*,*,#7702,.F.);
#11348=ORIENTED_EDGE('',*,*,#7703,.F.);
#11349=ORIENTED_EDGE('',*,*,#7704,.T.);
#11350=ORIENTED_EDGE('',*,*,#7705,.F.);
#11351=ORIENTED_EDGE('',*,*,#7706,.F.);
#11352=ORIENTED_EDGE('',*,*,#7696,.T.);
#11353=ORIENTED_EDGE('',*,*,#7704,.F.);
#11354=ORIENTED_EDGE('',*,*,#7676,.F.);
#11355=ORIENTED_EDGE('',*,*,#7706,.T.);
#11356=ORIENTED_EDGE('',*,*,#7707,.F.);
#11357=ORIENTED_EDGE('',*,*,#7708,.F.);
#11358=ORIENTED_EDGE('',*,*,#7707,.T.);
#11359=ORIENTED_EDGE('',*,*,#7705,.T.);
#11360=ORIENTED_EDGE('',*,*,#7703,.T.);
#11361=ORIENTED_EDGE('',*,*,#7709,.T.);
#11362=ORIENTED_EDGE('',*,*,#7710,.F.);
#11363=ORIENTED_EDGE('',*,*,#7711,.T.);
#11364=ORIENTED_EDGE('',*,*,#7712,.F.);
#11365=ORIENTED_EDGE('',*,*,#7713,.T.);
#11366=ORIENTED_EDGE('',*,*,#7714,.T.);
#11367=ORIENTED_EDGE('',*,*,#7715,.T.);
#11368=ORIENTED_EDGE('',*,*,#7709,.F.);
#11369=ORIENTED_EDGE('',*,*,#7702,.T.);
#11370=ORIENTED_EDGE('',*,*,#7684,.F.);
#11371=ORIENTED_EDGE('',*,*,#7716,.F.);
#11372=ORIENTED_EDGE('',*,*,#7713,.F.);
#11373=ORIENTED_EDGE('',*,*,#7717,.F.);
#11374=ORIENTED_EDGE('',*,*,#7679,.F.);
#11375=ORIENTED_EDGE('',*,*,#7718,.F.);
#11376=ORIENTED_EDGE('',*,*,#7719,.F.);
#11377=ORIENTED_EDGE('',*,*,#7682,.F.);
#11378=ORIENTED_EDGE('',*,*,#7720,.F.);
#11379=ORIENTED_EDGE('',*,*,#7711,.F.);
#11380=ORIENTED_EDGE('',*,*,#7721,.T.);
#11381=ORIENTED_EDGE('',*,*,#7716,.T.);
#11382=ORIENTED_EDGE('',*,*,#7683,.F.);
#11383=ORIENTED_EDGE('',*,*,#7719,.T.);
#11384=ORIENTED_EDGE('',*,*,#7722,.F.);
#11385=ORIENTED_EDGE('',*,*,#7723,.F.);
#11386=ORIENTED_EDGE('',*,*,#7677,.F.);
#11387=ORIENTED_EDGE('',*,*,#7708,.T.);
#11388=ORIENTED_EDGE('',*,*,#7715,.F.);
#11389=ORIENTED_EDGE('',*,*,#7724,.T.);
#11390=ORIENTED_EDGE('',*,*,#7718,.T.);
#11391=ORIENTED_EDGE('',*,*,#7678,.F.);
#11392=ORIENTED_EDGE('',*,*,#7723,.T.);
#11393=ORIENTED_EDGE('',*,*,#7710,.T.);
#11394=ORIENTED_EDGE('',*,*,#7721,.F.);
#11395=ORIENTED_EDGE('',*,*,#7722,.T.);
#11396=ORIENTED_EDGE('',*,*,#7725,.T.);
#11397=ORIENTED_EDGE('',*,*,#7670,.F.);
#11398=ORIENTED_EDGE('',*,*,#7688,.T.);
#11399=ORIENTED_EDGE('',*,*,#7694,.F.);
#11400=ORIENTED_EDGE('',*,*,#7726,.T.);
#11401=ORIENTED_EDGE('',*,*,#7725,.F.);
#11402=ORIENTED_EDGE('',*,*,#7727,.T.);
#11403=ORIENTED_EDGE('',*,*,#7728,.F.);
#11404=ORIENTED_EDGE('',*,*,#7729,.F.);
#11405=ORIENTED_EDGE('',*,*,#7730,.T.);
#11406=ORIENTED_EDGE('',*,*,#7731,.T.);
#11407=ORIENTED_EDGE('',*,*,#7730,.F.);
#11408=ORIENTED_EDGE('',*,*,#7732,.F.);
#11409=ORIENTED_EDGE('',*,*,#7727,.F.);
#11410=ORIENTED_EDGE('',*,*,#7733,.F.);
#11411=ORIENTED_EDGE('',*,*,#7643,.T.);
#11412=ORIENTED_EDGE('',*,*,#7733,.T.);
#11413=ORIENTED_EDGE('',*,*,#7734,.T.);
#11414=ORIENTED_EDGE('',*,*,#7735,.F.);
#11415=ORIENTED_EDGE('',*,*,#7734,.F.);
#11416=ORIENTED_EDGE('',*,*,#7728,.T.);
#11417=ORIENTED_EDGE('',*,*,#7732,.T.);
#11418=ORIENTED_EDGE('',*,*,#7729,.T.);
#11419=ORIENTED_EDGE('',*,*,#7736,.F.);
#11420=ORIENTED_EDGE('',*,*,#7735,.T.);
#11421=ORIENTED_EDGE('',*,*,#7640,.T.);
#11422=ORIENTED_EDGE('',*,*,#7637,.T.);
#11423=ORIENTED_EDGE('',*,*,#7634,.T.);
#11424=ORIENTED_EDGE('',*,*,#7631,.T.);
#11425=ORIENTED_EDGE('',*,*,#7736,.T.);
#11426=ORIENTED_EDGE('',*,*,#7737,.T.);
#11427=ORIENTED_EDGE('',*,*,#7680,.F.);
#11428=ORIENTED_EDGE('',*,*,#7717,.T.);
#11429=ORIENTED_EDGE('',*,*,#7712,.T.);
#11430=ORIENTED_EDGE('',*,*,#7720,.T.);
#11431=ORIENTED_EDGE('',*,*,#7681,.F.);
#11432=ORIENTED_EDGE('',*,*,#7737,.F.);
#11433=ORIENTED_EDGE('',*,*,#7714,.F.);
#11434=ORIENTED_EDGE('',*,*,#7724,.F.);
#11435=ORIENTED_EDGE('',*,*,#7646,.T.);
#11436=ORIENTED_EDGE('',*,*,#7649,.T.);
#11437=ORIENTED_EDGE('',*,*,#7652,.T.);
#11438=ORIENTED_EDGE('',*,*,#7731,.F.);
#11439=ORIENTED_EDGE('',*,*,#7667,.F.);
#11440=ORIENTED_EDGE('',*,*,#7726,.F.);
#11441=ORIENTED_EDGE('',*,*,#7693,.F.);
#11442=ORIENTED_EDGE('',*,*,#7698,.T.);
#11443=ORIENTED_EDGE('',*,*,#7699,.F.);
#11444=ORIENTED_EDGE('',*,*,#7701,.T.);
#11445=ORIENTED_EDGE('',*,*,#7691,.F.);
#11446=ORIENTED_EDGE('',*,*,#7689,.T.);
#11447=ORIENTED_EDGE('',*,*,#7645,.T.);
#11448=ORIENTED_EDGE('',*,*,#7657,.T.);
#11449=ORIENTED_EDGE('',*,*,#7660,.T.);
#11450=ORIENTED_EDGE('',*,*,#7663,.T.);
#11451=ORIENTED_EDGE('',*,*,#7666,.T.);
#12251=CYLINDRICAL_SURFACE('',#13877,1.);
#12252=CYLINDRICAL_SURFACE('',#13881,1.);
#12253=CYLINDRICAL_SURFACE('',#13885,1.);
#12254=CYLINDRICAL_SURFACE('',#13889,1.);
#12255=CYLINDRICAL_SURFACE('',#13893,8.5);
#12256=CYLINDRICAL_SURFACE('',#13896,1.);
#12257=CYLINDRICAL_SURFACE('',#13900,1.);
#12258=CYLINDRICAL_SURFACE('',#13904,1.);
#12259=CYLINDRICAL_SURFACE('',#13908,2.5);
#12260=CYLINDRICAL_SURFACE('',#13911,2.5);
#12261=CYLINDRICAL_SURFACE('',#13914,2.5);
#12262=CYLINDRICAL_SURFACE('',#13917,2.5);
#12263=CYLINDRICAL_SURFACE('',#13920,5.);
#12264=CYLINDRICAL_SURFACE('',#13930,5.);
#12265=CYLINDRICAL_SURFACE('',#13932,5.);
#12266=CYLINDRICAL_SURFACE('',#13935,5.);
#12267=CYLINDRICAL_SURFACE('',#13943,13.5);
#12268=CYLINDRICAL_SURFACE('',#13960,10.5);
#12269=CYLINDRICAL_SURFACE('',#13964,20.);
#12270=CYLINDRICAL_SURFACE('',#13968,23.);
#12786=ADVANCED_FACE('',(#1256),#12251,.F.);
#12787=ADVANCED_FACE('',(#1257),#525,.T.);
#12788=ADVANCED_FACE('',(#1258),#12252,.F.);
#12789=ADVANCED_FACE('',(#1259),#526,.T.);
#12790=ADVANCED_FACE('',(#1260),#12253,.F.);
#12791=ADVANCED_FACE('',(#1261),#527,.T.);
#12792=ADVANCED_FACE('',(#1262),#12254,.F.);
#12793=ADVANCED_FACE('',(#1263),#528,.T.);
#12794=ADVANCED_FACE('',(#1264),#12255,.F.);
#12795=ADVANCED_FACE('',(#1265),#12256,.F.);
#12796=ADVANCED_FACE('',(#1266),#529,.T.);
#12797=ADVANCED_FACE('',(#1267),#12257,.F.);
#12798=ADVANCED_FACE('',(#1268),#530,.T.);
#12799=ADVANCED_FACE('',(#1269),#12258,.F.);
#12800=ADVANCED_FACE('',(#1270),#531,.T.);
#12801=ADVANCED_FACE('',(#1271),#12259,.F.);
#12802=ADVANCED_FACE('',(#1272),#12260,.F.);
#12803=ADVANCED_FACE('',(#1273),#12261,.F.);
#12804=ADVANCED_FACE('',(#1274),#12262,.F.);
#12805=ADVANCED_FACE('',(#1275),#12263,.T.);
#12806=ADVANCED_FACE('',(#1276,#378,#379,#380,#381),#532,.T.);
#12807=ADVANCED_FACE('',(#1277),#533,.T.);
#12808=ADVANCED_FACE('',(#1278),#12264,.T.);
#12809=ADVANCED_FACE('',(#1279),#12265,.T.);
#12810=ADVANCED_FACE('',(#1280),#534,.T.);
#12811=ADVANCED_FACE('',(#1281),#12266,.T.);
#12812=ADVANCED_FACE('',(#1282),#535,.T.);
#12813=ADVANCED_FACE('',(#1283),#536,.F.);
#12814=ADVANCED_FACE('',(#1284),#537,.T.);
#12815=ADVANCED_FACE('',(#1285),#538,.T.);
#12816=ADVANCED_FACE('',(#1286),#12267,.T.);
#12817=ADVANCED_FACE('',(#1287),#539,.T.);
#12818=ADVANCED_FACE('',(#1288),#540,.T.);
#12819=ADVANCED_FACE('',(#1289),#541,.T.);
#12820=ADVANCED_FACE('',(#1290),#542,.F.);
#12821=ADVANCED_FACE('',(#1291),#543,.T.);
#12822=ADVANCED_FACE('',(#1292),#544,.T.);
#12823=ADVANCED_FACE('',(#1293,#382),#545,.F.);
#12824=ADVANCED_FACE('',(#1294),#546,.F.);
#12825=ADVANCED_FACE('',(#1295),#12268,.F.);
#12826=ADVANCED_FACE('',(#1296,#383),#547,.T.);
#12827=ADVANCED_FACE('',(#1297,#384),#12269,.F.);
#12828=ADVANCED_FACE('',(#1298,#385,#386,#387,#388,#389),#548,.T.);
#12829=ADVANCED_FACE('',(#1299),#12270,.T.);
#12830=ADVANCED_FACE('',(#1300,#390,#391,#392,#393),#549,.T.);
#12831=ADVANCED_FACE('',(#1301,#394,#395,#396,#397,#398),#550,.T.);
#12997=CLOSED_SHELL('',(#12786,#12787,#12788,#12789,#12790,#12791,#12792,
#12793,#12794,#12795,#12796,#12797,#12798,#12799,#12800,#12801,#12802,#12803,
#12804,#12805,#12806,#12807,#12808,#12809,#12810,#12811,#12812,#12813,#12814,
#12815,#12816,#12817,#12818,#12819,#12820,#12821,#12822,#12823,#12824,#12825,
#12826,#12827,#12828,#12829,#12830,#12831));
#13876=AXIS2_PLACEMENT_3D('',#87129,#16236,#16237);
#13877=AXIS2_PLACEMENT_3D('',#87130,#16238,#16239);
#13878=AXIS2_PLACEMENT_3D('',#87132,#16240,#16241);
#13879=AXIS2_PLACEMENT_3D('',#87135,#16243,#16244);
#13880=AXIS2_PLACEMENT_3D('',#87136,#16245,#16246);
#13881=AXIS2_PLACEMENT_3D('',#87137,#16247,#16248);
#13882=AXIS2_PLACEMENT_3D('',#87139,#16249,#16250);
#13883=AXIS2_PLACEMENT_3D('',#87142,#16252,#16253);
#13884=AXIS2_PLACEMENT_3D('',#87143,#16254,#16255);
#13885=AXIS2_PLACEMENT_3D('',#87144,#16256,#16257);
#13886=AXIS2_PLACEMENT_3D('',#87146,#16258,#16259);
#13887=AXIS2_PLACEMENT_3D('',#87149,#16261,#16262);
#13888=AXIS2_PLACEMENT_3D('',#87150,#16263,#16264);
#13889=AXIS2_PLACEMENT_3D('',#87151,#16265,#16266);
#13890=AXIS2_PLACEMENT_3D('',#87153,#16267,#16268);
#13891=AXIS2_PLACEMENT_3D('',#87156,#16270,#16271);
#13892=AXIS2_PLACEMENT_3D('',#87157,#16272,#16273);
#13893=AXIS2_PLACEMENT_3D('',#87158,#16274,#16275);
#13894=AXIS2_PLACEMENT_3D('',#87160,#16276,#16277);
#13895=AXIS2_PLACEMENT_3D('',#87163,#16279,#16280);
#13896=AXIS2_PLACEMENT_3D('',#87164,#16281,#16282);
#13897=AXIS2_PLACEMENT_3D('',#87166,#16283,#16284);
#13898=AXIS2_PLACEMENT_3D('',#87169,#16286,#16287);
#13899=AXIS2_PLACEMENT_3D('',#87170,#16288,#16289);
#13900=AXIS2_PLACEMENT_3D('',#87171,#16290,#16291);
#13901=AXIS2_PLACEMENT_3D('',#87173,#16292,#16293);
#13902=AXIS2_PLACEMENT_3D('',#87176,#16295,#16296);
#13903=AXIS2_PLACEMENT_3D('',#87177,#16297,#16298);
#13904=AXIS2_PLACEMENT_3D('',#87178,#16299,#16300);
#13905=AXIS2_PLACEMENT_3D('',#87180,#16301,#16302);
#13906=AXIS2_PLACEMENT_3D('',#87183,#16304,#16305);
#13907=AXIS2_PLACEMENT_3D('',#87184,#16306,#16307);
#13908=AXIS2_PLACEMENT_3D('',#87185,#16308,#16309);
#13909=AXIS2_PLACEMENT_3D('',#87187,#16310,#16311);
#13910=AXIS2_PLACEMENT_3D('',#87190,#16313,#16314);
#13911=AXIS2_PLACEMENT_3D('',#87191,#16315,#16316);
#13912=AXIS2_PLACEMENT_3D('',#87193,#16317,#16318);
#13913=AXIS2_PLACEMENT_3D('',#87196,#16320,#16321);
#13914=AXIS2_PLACEMENT_3D('',#87197,#16322,#16323);
#13915=AXIS2_PLACEMENT_3D('',#87199,#16324,#16325);
#13916=AXIS2_PLACEMENT_3D('',#87202,#16327,#16328);
#13917=AXIS2_PLACEMENT_3D('',#87203,#16329,#16330);
#13918=AXIS2_PLACEMENT_3D('',#87205,#16331,#16332);
#13919=AXIS2_PLACEMENT_3D('',#87208,#16334,#16335);
#13920=AXIS2_PLACEMENT_3D('',#87209,#16336,#16337);
#13921=AXIS2_PLACEMENT_3D('',#87212,#16338,#16339);
#13922=AXIS2_PLACEMENT_3D('',#87216,#16341,#16342);
#13923=AXIS2_PLACEMENT_3D('',#87218,#16344,#16345);
#13924=AXIS2_PLACEMENT_3D('',#87222,#16347,#16348);
#13925=AXIS2_PLACEMENT_3D('',#87226,#16350,#16351);
#13926=AXIS2_PLACEMENT_3D('',#87238,#16357,#16358);
#13927=AXIS2_PLACEMENT_3D('',#87240,#16359,#16360);
#13928=AXIS2_PLACEMENT_3D('',#87252,#16366,#16367);
#13929=AXIS2_PLACEMENT_3D('',#87254,#16369,#16370);
#13930=AXIS2_PLACEMENT_3D('',#87258,#16373,#16374);
#13931=AXIS2_PLACEMENT_3D('',#87260,#16375,#16376);
#13932=AXIS2_PLACEMENT_3D('',#87262,#16378,#16379);
#13933=AXIS2_PLACEMENT_3D('',#87265,#16380,#16381);
#13934=AXIS2_PLACEMENT_3D('',#87268,#16384,#16385);
#13935=AXIS2_PLACEMENT_3D('',#87273,#16389,#16390);
#13936=AXIS2_PLACEMENT_3D('',#87275,#16391,#16392);
#13937=AXIS2_PLACEMENT_3D('',#87277,#16394,#16395);
#13938=AXIS2_PLACEMENT_3D('',#87279,#16397,#16398);
#13939=AXIS2_PLACEMENT_3D('',#87283,#16400,#16401);
#13940=AXIS2_PLACEMENT_3D('',#87285,#16403,#16404);
#13941=AXIS2_PLACEMENT_3D('',#87289,#16407,#16408);
#13942=AXIS2_PLACEMENT_3D('',#87291,#16409,#16410);
#13943=AXIS2_PLACEMENT_3D('',#87293,#16412,#16413);
#13944=AXIS2_PLACEMENT_3D('',#87297,#16415,#16416);
#13945=AXIS2_PLACEMENT_3D('',#87363,#16419,#16420);
#13946=AXIS2_PLACEMENT_3D('',#87365,#16422,#16423);
#13947=AXIS2_PLACEMENT_3D('',#87367,#16425,#16426);
#13948=AXIS2_PLACEMENT_3D('',#87368,#16427,#16428);
#13949=AXIS2_PLACEMENT_3D('',#87370,#16430,#16431);
#13950=AXIS2_PLACEMENT_3D('',#87372,#16433,#16434);
#13951=AXIS2_PLACEMENT_3D('',#87373,#16435,#16436);
#13952=AXIS2_PLACEMENT_3D('',#87375,#16437,#16438);
#13953=AXIS2_PLACEMENT_3D('',#87376,#16439,#16440);
#13954=AXIS2_PLACEMENT_3D('',#87377,#16441,#16442);
#13955=AXIS2_PLACEMENT_3D('',#87379,#16444,#16445);
#13956=AXIS2_PLACEMENT_3D('',#87380,#16446,#16447);
#13957=AXIS2_PLACEMENT_3D('',#87381,#16448,#16449);
#13958=AXIS2_PLACEMENT_3D('',#87383,#16450,#16451);
#13959=AXIS2_PLACEMENT_3D('',#87384,#16452,#16453);
#13960=AXIS2_PLACEMENT_3D('',#87386,#16455,#16456);
#13961=AXIS2_PLACEMENT_3D('',#87421,#16459,#16460);
#13962=AXIS2_PLACEMENT_3D('',#87449,#16461,#16462);
#13963=AXIS2_PLACEMENT_3D('',#87451,#16463,#16464);
#13964=AXIS2_PLACEMENT_3D('',#87452,#16465,#16466);
#13965=AXIS2_PLACEMENT_3D('',#87455,#16468,#16469);
#13966=AXIS2_PLACEMENT_3D('',#87456,#16470,#16471);
#13967=AXIS2_PLACEMENT_3D('',#87458,#16472,#16473);
#13968=AXIS2_PLACEMENT_3D('',#87459,#16474,#16475);
#13969=AXIS2_PLACEMENT_3D('',#87461,#16477,#16478);
#13970=AXIS2_PLACEMENT_3D('',#87462,#16479,#16480);
#16236=DIRECTION('axis',(0.,0.,1.));
#16237=DIRECTION('refdir',(1.,0.,0.));
#16238=DIRECTION('center_axis',(0.,0.,-1.));
#16239=DIRECTION('ref_axis',(-1.,0.,0.));
#16240=DIRECTION('center_axis',(0.,0.,-1.));
#16241=DIRECTION('ref_axis',(-1.,0.,0.));
#16242=DIRECTION('',(0.,0.,-1.));
#16243=DIRECTION('center_axis',(0.,0.,-1.));
#16244=DIRECTION('ref_axis',(-1.,0.,0.));
#16245=DIRECTION('center_axis',(0.,0.,1.));
#16246=DIRECTION('ref_axis',(-1.,0.,0.));
#16247=DIRECTION('center_axis',(0.,0.,-1.));
#16248=DIRECTION('ref_axis',(-1.,0.,0.));
#16249=DIRECTION('center_axis',(0.,0.,-1.));
#16250=DIRECTION('ref_axis',(-1.,0.,0.));
#16251=DIRECTION('',(0.,0.,-1.));
#16252=DIRECTION('center_axis',(0.,0.,-1.));
#16253=DIRECTION('ref_axis',(-1.,0.,0.));
#16254=DIRECTION('center_axis',(0.,0.,1.));
#16255=DIRECTION('ref_axis',(-1.,0.,0.));
#16256=DIRECTION('center_axis',(0.,0.,-1.));
#16257=DIRECTION('ref_axis',(-1.,0.,0.));
#16258=DIRECTION('center_axis',(0.,0.,-1.));
#16259=DIRECTION('ref_axis',(-1.,0.,0.));
#16260=DIRECTION('',(0.,0.,-1.));
#16261=DIRECTION('center_axis',(0.,0.,-1.));
#16262=DIRECTION('ref_axis',(-1.,0.,0.));
#16263=DIRECTION('center_axis',(0.,0.,1.));
#16264=DIRECTION('ref_axis',(-1.,0.,0.));
#16265=DIRECTION('center_axis',(0.,0.,-1.));
#16266=DIRECTION('ref_axis',(-1.,0.,0.));
#16267=DIRECTION('center_axis',(0.,0.,-1.));
#16268=DIRECTION('ref_axis',(-1.,0.,0.));
#16269=DIRECTION('',(0.,0.,-1.));
#16270=DIRECTION('center_axis',(0.,0.,-1.));
#16271=DIRECTION('ref_axis',(-1.,0.,0.));
#16272=DIRECTION('center_axis',(0.,0.,1.));
#16273=DIRECTION('ref_axis',(-1.,0.,0.));
#16274=DIRECTION('center_axis',(0.,0.,-1.));
#16275=DIRECTION('ref_axis',(-1.,0.,0.));
#16276=DIRECTION('center_axis',(0.,0.,-1.));
#16277=DIRECTION('ref_axis',(-1.,0.,0.));
#16278=DIRECTION('',(0.,0.,-1.));
#16279=DIRECTION('center_axis',(0.,0.,1.));
#16280=DIRECTION('ref_axis',(-1.,0.,0.));
#16281=DIRECTION('center_axis',(-1.,0.,0.));
#16282=DIRECTION('ref_axis',(0.,1.,0.));
#16283=DIRECTION('center_axis',(-1.,0.,0.));
#16284=DIRECTION('ref_axis',(0.,1.,0.));
#16285=DIRECTION('',(-1.,0.,0.));
#16286=DIRECTION('center_axis',(-1.,0.,0.));
#16287=DIRECTION('ref_axis',(0.,1.,0.));
#16288=DIRECTION('center_axis',(1.,0.,0.));
#16289=DIRECTION('ref_axis',(0.,1.,0.));
#16290=DIRECTION('center_axis',(-1.,0.,0.));
#16291=DIRECTION('ref_axis',(0.,1.,0.));
#16292=DIRECTION('center_axis',(-1.,0.,0.));
#16293=DIRECTION('ref_axis',(0.,1.,0.));
#16294=DIRECTION('',(-1.,0.,0.));
#16295=DIRECTION('center_axis',(-1.,0.,0.));
#16296=DIRECTION('ref_axis',(0.,1.,0.));
#16297=DIRECTION('center_axis',(1.,0.,0.));
#16298=DIRECTION('ref_axis',(0.,1.,0.));
#16299=DIRECTION('center_axis',(-1.,0.,0.));
#16300=DIRECTION('ref_axis',(0.,1.,0.));
#16301=DIRECTION('center_axis',(-1.,0.,0.));
#16302=DIRECTION('ref_axis',(0.,1.,0.));
#16303=DIRECTION('',(-1.,0.,0.));
#16304=DIRECTION('center_axis',(-1.,0.,0.));
#16305=DIRECTION('ref_axis',(0.,1.,0.));
#16306=DIRECTION('center_axis',(1.,0.,0.));
#16307=DIRECTION('ref_axis',(0.,1.,0.));
#16308=DIRECTION('center_axis',(0.,0.,-1.));
#16309=DIRECTION('ref_axis',(-1.,0.,0.));
#16310=DIRECTION('center_axis',(0.,0.,-1.));
#16311=DIRECTION('ref_axis',(-1.,0.,0.));
#16312=DIRECTION('',(0.,0.,-1.));
#16313=DIRECTION('center_axis',(0.,0.,1.));
#16314=DIRECTION('ref_axis',(-1.,0.,0.));
#16315=DIRECTION('center_axis',(0.,0.,-1.));
#16316=DIRECTION('ref_axis',(-1.,0.,0.));
#16317=DIRECTION('center_axis',(0.,0.,-1.));
#16318=DIRECTION('ref_axis',(-1.,0.,0.));
#16319=DIRECTION('',(0.,0.,-1.));
#16320=DIRECTION('center_axis',(0.,0.,1.));
#16321=DIRECTION('ref_axis',(-1.,0.,0.));
#16322=DIRECTION('center_axis',(0.,0.,-1.));
#16323=DIRECTION('ref_axis',(-1.,0.,0.));
#16324=DIRECTION('center_axis',(0.,0.,-1.));
#16325=DIRECTION('ref_axis',(-1.,0.,0.));
#16326=DIRECTION('',(0.,0.,-1.));
#16327=DIRECTION('center_axis',(0.,0.,1.));
#16328=DIRECTION('ref_axis',(-1.,0.,0.));
#16329=DIRECTION('center_axis',(0.,0.,-1.));
#16330=DIRECTION('ref_axis',(-1.,0.,0.));
#16331=DIRECTION('center_axis',(0.,0.,-1.));
#16332=DIRECTION('ref_axis',(-1.,0.,0.));
#16333=DIRECTION('',(0.,0.,-1.));
#16334=DIRECTION('center_axis',(0.,0.,1.));
#16335=DIRECTION('ref_axis',(-1.,0.,0.));
#16336=DIRECTION('center_axis',(0.,0.,-1.));
#16337=DIRECTION('ref_axis',(-0.707106781186548,-0.707106781186548,0.));
#16338=DIRECTION('center_axis',(0.,0.,1.));
#16339=DIRECTION('ref_axis',(-0.707106781186548,-0.707106781186548,0.));
#16340=DIRECTION('',(0.,0.,1.));
#16341=DIRECTION('center_axis',(0.,0.,-1.));
#16342=DIRECTION('ref_axis',(-0.707106781186548,-0.707106781186548,0.));
#16343=DIRECTION('',(0.,0.,-1.));
#16344=DIRECTION('center_axis',(0.,0.,1.));
#16345=DIRECTION('ref_axis',(-1.,0.,0.));
#16346=DIRECTION('',(1.,0.,0.));
#16347=DIRECTION('center_axis',(0.,0.,-1.));
#16348=DIRECTION('ref_axis',(0.707106781186548,-0.707106781186548,0.));
#16349=DIRECTION('',(-1.11022302462516E-16,1.,0.));
#16350=DIRECTION('center_axis',(0.,0.,-1.));
#16351=DIRECTION('ref_axis',(0.707106781186548,0.707106781186548,0.));
#16352=DIRECTION('',(-1.,0.,0.));
#16353=DIRECTION('',(0.,-1.,0.));
#16354=DIRECTION('',(1.,0.,0.));
#16355=DIRECTION('',(0.,-1.,0.));
#16356=DIRECTION('',(-1.,0.,0.));
#16357=DIRECTION('center_axis',(0.,0.,-1.));
#16358=DIRECTION('ref_axis',(1.,0.,0.));
#16359=DIRECTION('center_axis',(0.,0.,-1.));
#16360=DIRECTION('ref_axis',(1.,0.,0.));
#16361=DIRECTION('',(-1.,0.,0.));
#16362=DIRECTION('',(0.,1.,0.));
#16363=DIRECTION('',(1.,0.,0.));
#16364=DIRECTION('',(0.,1.,0.));
#16365=DIRECTION('',(-1.,0.,0.));
#16366=DIRECTION('center_axis',(0.,0.,-1.));
#16367=DIRECTION('ref_axis',(-0.707106781186548,0.707106781186548,0.));
#16368=DIRECTION('',(1.11022302462516E-16,1.,0.));
#16369=DIRECTION('center_axis',(0.,-1.,0.));
#16370=DIRECTION('ref_axis',(-1.,0.,0.));
#16371=DIRECTION('',(-1.,0.,0.));
#16372=DIRECTION('',(0.,0.,-1.));
#16373=DIRECTION('center_axis',(0.,0.,-1.));
#16374=DIRECTION('ref_axis',(0.707106781186548,-0.707106781186548,0.));
#16375=DIRECTION('center_axis',(0.,0.,1.));
#16376=DIRECTION('ref_axis',(0.707106781186548,-0.707106781186548,0.));
#16377=DIRECTION('',(0.,0.,1.));
#16378=DIRECTION('center_axis',(0.,0.,-1.));
#16379=DIRECTION('ref_axis',(-0.707106781186548,0.707106781186548,0.));
#16380=DIRECTION('center_axis',(0.,0.,1.));
#16381=DIRECTION('ref_axis',(-0.707106781186548,0.707106781186548,0.));
#16382=DIRECTION('',(0.,0.,1.));
#16383=DIRECTION('',(0.,0.,-1.));
#16384=DIRECTION('center_axis',(0.,1.,0.));
#16385=DIRECTION('ref_axis',(1.,0.,0.));
#16386=DIRECTION('',(-1.,0.,0.));
#16387=DIRECTION('',(0.,0.,1.));
#16388=DIRECTION('',(1.,0.,0.));
#16389=DIRECTION('center_axis',(0.,0.,-1.));
#16390=DIRECTION('ref_axis',(0.707106781186548,0.707106781186548,0.));
#16391=DIRECTION('center_axis',(0.,0.,1.));
#16392=DIRECTION('ref_axis',(0.707106781186548,0.707106781186548,0.));
#16393=DIRECTION('',(0.,0.,-1.));
#16394=DIRECTION('center_axis',(1.,1.11022302462516E-16,0.));
#16395=DIRECTION('ref_axis',(1.11022302462516E-16,-1.,0.));
#16396=DIRECTION('',(1.11022302462516E-16,-1.,0.));
#16397=DIRECTION('center_axis',(1.,0.,0.));
#16398=DIRECTION('ref_axis',(0.,1.,0.));
#16399=DIRECTION('',(0.,0.342020143325669,-0.939692620785908));
#16400=DIRECTION('center_axis',(-1.,0.,0.));
#16401=DIRECTION('ref_axis',(0.,1.,0.));
#16402=DIRECTION('',(0.,0.447213595499958,-0.894427190999916));
#16403=DIRECTION('center_axis',(0.,0.894427190999916,0.447213595499958));
#16404=DIRECTION('ref_axis',(0.,-0.447213595499958,0.894427190999916));
#16405=DIRECTION('',(-1.,0.,0.));
#16406=DIRECTION('',(0.,-0.447213595499958,0.894427190999916));
#16407=DIRECTION('center_axis',(1.,0.,0.));
#16408=DIRECTION('ref_axis',(0.,1.,0.));
#16409=DIRECTION('center_axis',(1.,0.,0.));
#16410=DIRECTION('ref_axis',(0.,1.,0.));
#16411=DIRECTION('',(0.,-0.342020143325669,0.939692620785908));
#16412=DIRECTION('center_axis',(1.,0.,0.));
#16413=DIRECTION('ref_axis',(0.,-3.82856869892695E-16,1.));
#16414=DIRECTION('',(-1.,0.,0.));
#16415=DIRECTION('center_axis',(-1.,0.,0.));
#16416=DIRECTION('ref_axis',(0.,1.,0.));
#16417=DIRECTION('',(1.,0.,0.));
#16418=DIRECTION('',(1.,0.,0.));
#16419=DIRECTION('center_axis',(-1.,0.,0.));
#16420=DIRECTION('ref_axis',(0.,1.,0.));
#16421=DIRECTION('',(-1.,0.,0.));
#16422=DIRECTION('center_axis',(0.,0.939692620785908,0.342020143325669));
#16423=DIRECTION('ref_axis',(0.,-0.342020143325669,0.939692620785908));
#16424=DIRECTION('',(0.,0.342020143325669,-0.939692620785908));
#16425=DIRECTION('center_axis',(0.,-0.939692620785908,0.342020143325669));
#16426=DIRECTION('ref_axis',(0.,-0.342020143325669,-0.939692620785908));
#16427=DIRECTION('center_axis',(0.,0.939692620785908,-0.342020143325669));
#16428=DIRECTION('ref_axis',(0.,0.342020143325669,0.939692620785908));
#16429=DIRECTION('',(0.,-0.342020143325669,-0.939692620785908));
#16430=DIRECTION('center_axis',(0.,-0.939692620785908,0.342020143325669));
#16431=DIRECTION('ref_axis',(0.,-0.342020143325669,-0.939692620785908));
#16432=DIRECTION('',(0.,0.342020143325669,0.939692620785908));
#16433=DIRECTION('center_axis',(0.,0.939692620785908,-0.342020143325669));
#16434=DIRECTION('ref_axis',(0.,0.342020143325669,0.939692620785908));
#16435=DIRECTION('center_axis',(1.,0.,0.));
#16436=DIRECTION('ref_axis',(0.,1.,0.));
#16437=DIRECTION('center_axis',(1.,0.,0.));
#16438=DIRECTION('ref_axis',(0.,1.,0.));
#16439=DIRECTION('center_axis',(-1.,0.,0.));
#16440=DIRECTION('ref_axis',(0.,1.,0.));
#16441=DIRECTION('center_axis',(0.,0.939692620785908,0.342020143325669));
#16442=DIRECTION('ref_axis',(0.,-0.342020143325669,0.939692620785908));
#16443=DIRECTION('',(0.,-0.342020143325669,0.939692620785908));
#16444=DIRECTION('center_axis',(1.,0.,0.));
#16445=DIRECTION('ref_axis',(0.,1.,0.));
#16446=DIRECTION('center_axis',(-1.,0.,0.));
#16447=DIRECTION('ref_axis',(0.,-0.342020143325665,-0.93969262078591));
#16448=DIRECTION('center_axis',(1.,0.,0.));
#16449=DIRECTION('ref_axis',(0.,1.,0.));
#16450=DIRECTION('center_axis',(1.,0.,0.));
#16451=DIRECTION('ref_axis',(0.,1.,0.));
#16452=DIRECTION('center_axis',(1.,-1.11022302462516E-16,0.));
#16453=DIRECTION('ref_axis',(-1.11022302462516E-16,-1.,0.));
#16454=DIRECTION('',(-1.11022302462516E-16,-1.,0.));
#16455=DIRECTION('center_axis',(1.,0.,0.));
#16456=DIRECTION('ref_axis',(0.,1.,0.));
#16457=DIRECTION('',(1.,0.,0.));
#16458=DIRECTION('',(1.,0.,0.));
#16459=DIRECTION('center_axis',(1.,0.,0.));
#16460=DIRECTION('ref_axis',(0.,1.,0.));
#16461=DIRECTION('center_axis',(0.,0.,1.));
#16462=DIRECTION('ref_axis',(-1.,0.,0.));
#16463=DIRECTION('center_axis',(0.,0.,1.));
#16464=DIRECTION('ref_axis',(-1.,0.,0.));
#16465=DIRECTION('center_axis',(0.,0.,1.));
#16466=DIRECTION('ref_axis',(1.,0.,0.));
#16467=DIRECTION('',(0.,0.,1.));
#16468=DIRECTION('center_axis',(0.,0.,-1.));
#16469=DIRECTION('ref_axis',(1.,0.,0.));
#16470=DIRECTION('center_axis',(0.,0.,1.));
#16471=DIRECTION('ref_axis',(1.,0.,0.));
#16472=DIRECTION('center_axis',(0.,0.,-1.));
#16473=DIRECTION('ref_axis',(1.,0.,0.));
#16474=DIRECTION('center_axis',(0.,0.,1.));
#16475=DIRECTION('ref_axis',(1.,0.,0.));
#16476=DIRECTION('',(0.,0.,-1.));
#16477=DIRECTION('center_axis',(1.,0.,0.));
#16478=DIRECTION('ref_axis',(0.,1.,0.));
#16479=DIRECTION('center_axis',(0.,0.,-1.));
#16480=DIRECTION('ref_axis',(-1.,0.,0.));
#87129=CARTESIAN_POINT('',(0.,0.,0.));
#87130=CARTESIAN_POINT('Origin',(-21.3644359551636,4.74385774111043E-15,
30.0000004769));
#87131=CARTESIAN_POINT('',(-20.3644359551636,4.62139306119569E-15,27.0000004769));
#87132=CARTESIAN_POINT('Origin',(-21.3644359551636,4.74385774111043E-15,
27.0000004769));
#87133=CARTESIAN_POINT('',(-20.3644359551636,4.86632242102517E-15,22.0000004769));
#87134=CARTESIAN_POINT('',(-20.3644359551636,4.62139306119569E-15,30.0000004769));
#87135=CARTESIAN_POINT('Origin',(-21.3644359551636,4.74385774111043E-15,
22.0000004769));
#87136=CARTESIAN_POINT('Origin',(-21.3644359551636,4.71844785465692E-15,
22.0000004769));
#87137=CARTESIAN_POINT('Origin',(2.61638881080797E-15,21.3644359551636,
30.0000004769));
#87138=CARTESIAN_POINT('',(1.,21.3644359551636,27.0000004769));
#87139=CARTESIAN_POINT('Origin',(2.61638881080797E-15,21.3644359551636,
27.0000004769));
#87140=CARTESIAN_POINT('',(1.,21.3644359551636,22.0000004769));
#87141=CARTESIAN_POINT('',(1.,21.3644359551636,30.0000004769));
#87142=CARTESIAN_POINT('Origin',(2.61638881080797E-15,21.3644359551636,
22.0000004769));
#87143=CARTESIAN_POINT('Origin',(2.63677968348475E-15,21.3644359551636,
22.0000004769));
#87144=CARTESIAN_POINT('Origin',(0.,-21.3644359551636,30.0000004769));
#87145=CARTESIAN_POINT('',(1.,-21.3644359551636,27.0000004769));
#87146=CARTESIAN_POINT('Origin',(0.,-21.3644359551636,27.0000004769));
#87147=CARTESIAN_POINT('',(1.,-21.3644359551636,22.0000004769));
#87148=CARTESIAN_POINT('',(1.,-21.3644359551636,30.0000004769));
#87149=CARTESIAN_POINT('Origin',(0.,-21.3644359551636,22.0000004769));
#87150=CARTESIAN_POINT('Origin',(0.,-21.3644359551636,22.0000004769));
#87151=CARTESIAN_POINT('Origin',(21.3644359551636,4.74385774111043E-15,
30.0000004769));
#87152=CARTESIAN_POINT('',(22.3644359551636,4.62139306119569E-15,27.0000004769));
#87153=CARTESIAN_POINT('Origin',(21.3644359551636,4.74385774111043E-15,
27.0000004769));
#87154=CARTESIAN_POINT('',(22.3644359551636,4.86632242102517E-15,22.0000004769));
#87155=CARTESIAN_POINT('',(22.3644359551636,4.62139306119569E-15,30.0000004769));
#87156=CARTESIAN_POINT('Origin',(21.3644359551636,4.74385774111043E-15,
22.0000004769));
#87157=CARTESIAN_POINT('Origin',(21.3644359551636,4.71844785465692E-15,
22.0000004769));
#87158=CARTESIAN_POINT('Origin',(0.,0.,-27.));
#87159=CARTESIAN_POINT('',(8.5,1.04094977927525E-15,-27.));
#87160=CARTESIAN_POINT('Origin',(0.,0.,-27.));
#87161=CARTESIAN_POINT('',(8.5,1.04094977927525E-15,-28.));
#87162=CARTESIAN_POINT('',(8.5,-1.04094977927525E-15,-27.));
#87163=CARTESIAN_POINT('Origin',(0.,0.,-28.));
#87164=CARTESIAN_POINT('Origin',(26.3408711739,15.6090782051017,5.99920149541289));
#87165=CARTESIAN_POINT('',(23.3408711739,14.6090782051017,5.99920149541289));
#87166=CARTESIAN_POINT('Origin',(23.3408711739,15.6090782051017,5.99920149541289));
#87167=CARTESIAN_POINT('',(18.3408711739,14.6090782051017,5.99920149541289));
#87168=CARTESIAN_POINT('',(26.3408711739,14.6090782051017,5.99920149541289));
#87169=CARTESIAN_POINT('Origin',(18.3408711739,15.6090782051017,5.99920149541289));
#87170=CARTESIAN_POINT('Origin',(18.3408711739,15.6090782051017,5.99920149541289));
#87171=CARTESIAN_POINT('Origin',(26.3408711739,36.3909217948983,5.99920149541289));
#87172=CARTESIAN_POINT('',(23.3408711739,35.3909217948983,5.99920149541289));
#87173=CARTESIAN_POINT('Origin',(23.3408711739,36.3909217948983,5.99920149541289));
#87174=CARTESIAN_POINT('',(18.3408711739,35.3909217948983,5.99920149541289));
#87175=CARTESIAN_POINT('',(26.3408711739,35.3909217948983,5.99920149541289));
#87176=CARTESIAN_POINT('Origin',(18.3408711739,36.3909217948983,5.99920149541289));
#87177=CARTESIAN_POINT('Origin',(18.3408711739,36.3909217948983,5.99920149541289));
#87178=CARTESIAN_POINT('Origin',(26.3408711739,26.,-11.9984029908258));
#87179=CARTESIAN_POINT('',(23.3408711739,25.,-11.9984029908258));
#87180=CARTESIAN_POINT('Origin',(23.3408711739,26.,-11.9984029908258));
#87181=CARTESIAN_POINT('',(18.3408711739,25.,-11.9984029908258));
#87182=CARTESIAN_POINT('',(26.3408711739,25.,-11.9984029908258));
#87183=CARTESIAN_POINT('Origin',(18.3408711739,26.,-11.9984029908258));
#87184=CARTESIAN_POINT('Origin',(18.3408711739,26.,-11.9984029908258));
#87185=CARTESIAN_POINT('Origin',(25.,-24.,-23.));
#87186=CARTESIAN_POINT('',(27.5,-24.,-23.));
#87187=CARTESIAN_POINT('Origin',(25.,-24.,-23.));
#87188=CARTESIAN_POINT('',(27.5,-24.,-28.));
#87189=CARTESIAN_POINT('',(27.5,-24.,-23.));
#87190=CARTESIAN_POINT('Origin',(25.,-24.,-28.));
#87191=CARTESIAN_POINT('Origin',(25.,46.,-23.));
#87192=CARTESIAN_POINT('',(27.5,46.,-23.));
#87193=CARTESIAN_POINT('Origin',(25.,46.,-23.));
#87194=CARTESIAN_POINT('',(27.5,46.,-28.));
#87195=CARTESIAN_POINT('',(27.5,46.,-23.));
#87196=CARTESIAN_POINT('Origin',(25.,46.,-28.));
#87197=CARTESIAN_POINT('Origin',(-25.,-24.,-23.));
#87198=CARTESIAN_POINT('',(-22.5,-24.,-23.));
#87199=CARTESIAN_POINT('Origin',(-25.,-24.,-23.));
#87200=CARTESIAN_POINT('',(-22.5,-24.,-28.));
#87201=CARTESIAN_POINT('',(-22.5,-24.,-23.));
#87202=CARTESIAN_POINT('Origin',(-25.,-24.,-28.));
#87203=CARTESIAN_POINT('Origin',(-25.,46.,-23.));
#87204=CARTESIAN_POINT('',(-22.5,46.,-23.));
#87205=CARTESIAN_POINT('Origin',(-25.,46.,-23.));
#87206=CARTESIAN_POINT('',(-22.5,46.,-28.));
#87207=CARTESIAN_POINT('',(-22.5,46.,-23.));
#87208=CARTESIAN_POINT('Origin',(-25.,46.,-28.));
#87209=CARTESIAN_POINT('Origin',(-25.,-24.,-23.));
#87210=CARTESIAN_POINT('',(-30.,-24.,-28.));
#87211=CARTESIAN_POINT('',(-25.,-29.,-28.));
#87212=CARTESIAN_POINT('Origin',(-25.,-24.,-28.));
#87213=CARTESIAN_POINT('',(-25.,-29.,-23.));
#87214=CARTESIAN_POINT('',(-25.,-29.,-23.));
#87215=CARTESIAN_POINT('',(-30.,-24.,-23.));
#87216=CARTESIAN_POINT('Origin',(-25.,-24.,-23.));
#87217=CARTESIAN_POINT('',(-30.,-24.,-23.));
#87218=CARTESIAN_POINT('Origin',(0.,11.,-23.));
#87219=CARTESIAN_POINT('',(25.,-29.,-23.));
#87220=CARTESIAN_POINT('',(-30.,-29.,-23.));
#87221=CARTESIAN_POINT('',(30.,-24.,-23.));
#87222=CARTESIAN_POINT('Origin',(25.,-24.,-23.));
#87223=CARTESIAN_POINT('',(30.,46.,-23.));
#87224=CARTESIAN_POINT('',(30.,-29.,-23.));
#87225=CARTESIAN_POINT('',(25.,51.,-23.));
#87226=CARTESIAN_POINT('Origin',(25.,46.,-23.));
#87227=CARTESIAN_POINT('',(3.,51.,-23.));
#87228=CARTESIAN_POINT('',(30.,51.,-23.));
#87229=CARTESIAN_POINT('',(3.,34.3713153881227,-23.));
#87230=CARTESIAN_POINT('',(3.,25.9043179837241,-23.));
#87231=CARTESIAN_POINT('',(23.341,34.3713153881227,-23.));
#87232=CARTESIAN_POINT('',(0.,34.3713153881227,-23.));
#87233=CARTESIAN_POINT('',(23.341,17.6286846118773,-23.));
#87234=CARTESIAN_POINT('',(23.341,18.5,-23.));
#87235=CARTESIAN_POINT('',(14.7725921509309,17.6286846118481,-23.));
#87236=CARTESIAN_POINT('',(0.,17.6286846118773,-23.));
#87237=CARTESIAN_POINT('',(-23.,-2.81668763803891E-15,-23.0000000000237));
#87238=CARTESIAN_POINT('Origin',(0.,0.,-23.));
#87239=CARTESIAN_POINT('',(-14.7725921509309,17.6286846118481,-23.));
#87240=CARTESIAN_POINT('Origin',(0.,0.,-23.));
#87241=CARTESIAN_POINT('',(-23.341,17.6286846118773,-23.));
#87242=CARTESIAN_POINT('',(0.,17.6286846118773,-23.));
#87243=CARTESIAN_POINT('',(-23.341,34.3713153881227,-23.));
#87244=CARTESIAN_POINT('',(-23.341,18.5,-23.));
#87245=CARTESIAN_POINT('',(-3.,34.3713153881227,-23.));
#87246=CARTESIAN_POINT('',(0.,34.3713153881227,-23.));
#87247=CARTESIAN_POINT('',(-3.,51.,-23.));
#87248=CARTESIAN_POINT('',(-3.,25.9043179837241,-23.));
#87249=CARTESIAN_POINT('',(-25.,51.,-23.));
#87250=CARTESIAN_POINT('',(30.,51.,-23.));
#87251=CARTESIAN_POINT('',(-30.,46.,-23.));
#87252=CARTESIAN_POINT('Origin',(-25.,46.,-23.));
#87253=CARTESIAN_POINT('',(-30.,-29.,-23.));
#87254=CARTESIAN_POINT('Origin',(30.,-29.,-23.));
#87255=CARTESIAN_POINT('',(25.,-29.,-28.));
#87256=CARTESIAN_POINT('',(-30.,-29.,-28.));
#87257=CARTESIAN_POINT('',(25.,-29.,-23.));
#87258=CARTESIAN_POINT('Origin',(25.,-24.,-23.));
#87259=CARTESIAN_POINT('',(30.,-24.,-28.));
#87260=CARTESIAN_POINT('Origin',(25.,-24.,-28.));
#87261=CARTESIAN_POINT('',(30.,-24.,-23.));
#87262=CARTESIAN_POINT('Origin',(-25.,46.,-23.));
#87263=CARTESIAN_POINT('',(-25.,51.,-28.));
#87264=CARTESIAN_POINT('',(-30.,46.,-28.));
#87265=CARTESIAN_POINT('Origin',(-25.,46.,-28.));
#87266=CARTESIAN_POINT('',(-30.,46.,-23.));
#87267=CARTESIAN_POINT('',(-25.,51.,-23.));
#87268=CARTESIAN_POINT('Origin',(-30.,51.,-23.));
#87269=CARTESIAN_POINT('',(30.,51.,-23.));
#87270=CARTESIAN_POINT('',(25.,51.,-28.));
#87271=CARTESIAN_POINT('',(25.,51.,-23.));
#87272=CARTESIAN_POINT('',(30.,51.,-28.));
#87273=CARTESIAN_POINT('Origin',(25.,46.,-23.));
#87274=CARTESIAN_POINT('',(30.,46.,-28.));
#87275=CARTESIAN_POINT('Origin',(25.,46.,-28.));
#87276=CARTESIAN_POINT('',(30.,46.,-23.));
#87277=CARTESIAN_POINT('Origin',(30.,51.,-23.));
#87278=CARTESIAN_POINT('',(30.,-29.,-28.));
#87279=CARTESIAN_POINT('Origin',(-3.,40.8086359674483,-11.5));
#87280=CARTESIAN_POINT('',(-3.,30.6172719348965,-12.6858503806098));
#87281=CARTESIAN_POINT('',(-3.,32.8998127405133,-18.9570797030256));
#87282=CARTESIAN_POINT('',(-3.,39.5,0.));
#87283=CARTESIAN_POINT('Origin',(-3.,26.,7.77156117237612E-15));
#87284=CARTESIAN_POINT('',(-3.,39.5,9.86076131526265E-31));
#87285=CARTESIAN_POINT('Origin',(0.,51.,-23.));
#87286=CARTESIAN_POINT('',(3.,39.5,0.));
#87287=CARTESIAN_POINT('',(0.,39.5,1.11022302462516E-15));
#87288=CARTESIAN_POINT('',(3.,39.5,9.86076131526265E-31));
#87289=CARTESIAN_POINT('Origin',(3.,40.8086359674483,-11.5));
#87290=CARTESIAN_POINT('',(3.,30.6172719348965,-12.6858503806098));
#87291=CARTESIAN_POINT('Origin',(3.,26.,7.77156117237612E-15));
#87292=CARTESIAN_POINT('',(3.,32.8998127405133,-18.9570797030256));
#87293=CARTESIAN_POINT('Origin',(0.,26.,7.77156117237612E-15));
#87294=CARTESIAN_POINT('',(-23.341,30.6172719348965,-12.6858503806098));
#87295=CARTESIAN_POINT('',(0.,30.6172719348965,-12.6858503806098));
#87296=CARTESIAN_POINT('',(-23.3408711738295,21.3827280651035,-12.6858503806098));
#87297=CARTESIAN_POINT('Origin',(-23.3408711739,26.,7.77156117237612E-15));
#87298=CARTESIAN_POINT('',(-8.47224530415857,21.3827280651035,-12.6858503806098));
#87299=CARTESIAN_POINT('',(0.,21.3827280651035,-12.6858503806098));
#87300=CARTESIAN_POINT('',(8.47224530415857,21.3827280651035,-12.6858503806098));
#87301=CARTESIAN_POINT('Ctrl Pts',(-8.47224530415855,21.3827280651035,-12.6858503806098));
#87302=CARTESIAN_POINT('Ctrl Pts',(-9.35628286281192,21.0324554978147,-12.5583615922366));
#87303=CARTESIAN_POINT('Ctrl Pts',(-10.209624743653,20.6302930419102,-12.3957375602561));
#87304=CARTESIAN_POINT('Ctrl Pts',(-12.1079676069651,19.5944481184793,-11.9018501855925));
#87305=CARTESIAN_POINT('Ctrl Pts',(-13.1142232633922,18.928496485912,-11.5302951941811));
#87306=CARTESIAN_POINT('Ctrl Pts',(-14.6740782199554,17.7306523050959,-10.6891601041063));
#87307=CARTESIAN_POINT('Ctrl Pts',(-15.3466928743124,17.1509714206232,-10.226343468984));
#87308=CARTESIAN_POINT('Ctrl Pts',(-16.5328372723469,16.0106865238809,-9.11575746654458));
#87309=CARTESIAN_POINT('Ctrl Pts',(-17.0470433193552,15.4527028814967,-8.46602249011973));
#87310=CARTESIAN_POINT('Ctrl Pts',(-18.0617605062209,14.2705140920159,-6.79548401503536));
#87311=CARTESIAN_POINT('Ctrl Pts',(-18.5481190870437,13.6110072927135,-5.54965650514264));
#87312=CARTESIAN_POINT('Ctrl Pts',(-19.1670802823021,12.7245909828806,-2.83714766145209));
#87313=CARTESIAN_POINT('Ctrl Pts',(-19.3067345763078,12.5,-1.37132291257204));
#87314=CARTESIAN_POINT('Ctrl Pts',(-19.3067345763078,12.5,1.37132291257206));
#87315=CARTESIAN_POINT('Ctrl Pts',(-19.1670802823021,12.7245909828806,2.83714766145211));
#87316=CARTESIAN_POINT('Ctrl Pts',(-18.5481190870437,13.6110072927135,5.54965650514266));
#87317=CARTESIAN_POINT('Ctrl Pts',(-18.0617605062209,14.2705140920159,6.79548401503537));
#87318=CARTESIAN_POINT('Ctrl Pts',(-17.0470433193552,15.4527028814967,8.46602249011974));
#87319=CARTESIAN_POINT('Ctrl Pts',(-16.5328372723469,16.0106865238809,9.11575746654459));
#87320=CARTESIAN_POINT('Ctrl Pts',(-15.3466928743124,17.1509714206232,10.226343468984));
#87321=CARTESIAN_POINT('Ctrl Pts',(-14.6740782199554,17.7306523050959,10.6891601041063));
#87322=CARTESIAN_POINT('Ctrl Pts',(-13.1142232633922,18.928496485912,11.5302951941811));
#87323=CARTESIAN_POINT('Ctrl Pts',(-12.1079676069651,19.5944481184793,11.9018501855925));
#87324=CARTESIAN_POINT('Ctrl Pts',(-9.92554422303049,20.7853036940003,12.4696461176801));
#87325=CARTESIAN_POINT('Ctrl Pts',(-8.74955002586604,21.3099969687168,12.666995319975));
#87326=CARTESIAN_POINT('Ctrl Pts',(-6.30687367788335,22.1561289830517,12.9488785425586));
#87327=CARTESIAN_POINT('Ctrl Pts',(-5.03861971528053,22.4782166140122,13.0343544769648));
#87328=CARTESIAN_POINT('Ctrl Pts',(-2.49822268817386,22.9001483475584,13.141091066862));
#87329=CARTESIAN_POINT('Ctrl Pts',(-1.22608486406836,23.,13.1624465810882));
#87330=CARTESIAN_POINT('Ctrl Pts',(0.,23.,13.1624465810882));
#87331=CARTESIAN_POINT('Ctrl Pts',(1.22608486406836,23.,13.1624465810882));
#87332=CARTESIAN_POINT('Ctrl Pts',(2.49822268817386,22.9001483475584,13.141091066862));
#87333=CARTESIAN_POINT('Ctrl Pts',(5.03861971528053,22.4782166140122,13.0343544769648));
#87334=CARTESIAN_POINT('Ctrl Pts',(6.30687367788335,22.1561289830517,12.9488785425586));
#87335=CARTESIAN_POINT('Ctrl Pts',(8.74955002586604,21.3099969687168,12.666995319975));
#87336=CARTESIAN_POINT('Ctrl Pts',(9.92554422303049,20.7853036940003,12.4696461176801));
#87337=CARTESIAN_POINT('Ctrl Pts',(12.1079676069651,19.5944481184793,11.9018501855925));
#87338=CARTESIAN_POINT('Ctrl Pts',(13.1142232633922,18.928496485912,11.5302951941811));
#87339=CARTESIAN_POINT('Ctrl Pts',(14.6740782199554,17.7306523050959,10.6891601041063));
#87340=CARTESIAN_POINT('Ctrl Pts',(15.3466928743123,17.1509714206232,10.226343468984));
#87341=CARTESIAN_POINT('Ctrl Pts',(16.5328372723469,16.0106865238809,9.1157574665446));
#87342=CARTESIAN_POINT('Ctrl Pts',(17.0470433193552,15.4527028814967,8.46602249011975));
#87343=CARTESIAN_POINT('Ctrl Pts',(18.0617605062209,14.2705140920159,6.79548401503537));
#87344=CARTESIAN_POINT('Ctrl Pts',(18.5481190870437,13.6110072927135,5.54965650514266));
#87345=CARTESIAN_POINT('Ctrl Pts',(19.1670802823021,12.7245909828806,2.83714766145211));
#87346=CARTESIAN_POINT('Ctrl Pts',(19.3067345763078,12.5,1.37132291257206));
#87347=CARTESIAN_POINT('Ctrl Pts',(19.3067345763078,12.5,-1.37132291257204));
#87348=CARTESIAN_POINT('Ctrl Pts',(19.1670802823021,12.7245909828806,-2.83714766145209));
#87349=CARTESIAN_POINT('Ctrl Pts',(18.5481190870437,13.6110072927135,-5.54965650514264));
#87350=CARTESIAN_POINT('Ctrl Pts',(18.0617605062209,14.2705140920159,-6.79548401503536));
#87351=CARTESIAN_POINT('Ctrl Pts',(17.0470433193552,15.4527028814967,-8.46602249011973));
#87352=CARTESIAN_POINT('Ctrl Pts',(16.5328372723469,16.0106865238809,-9.11575746654458));
#87353=CARTESIAN_POINT('Ctrl Pts',(15.3466928743124,17.1509714206232,-10.226343468984));
#87354=CARTESIAN_POINT('Ctrl Pts',(14.6740782199554,17.7306523050959,-10.6891601041063));
#87355=CARTESIAN_POINT('Ctrl Pts',(13.1142232633922,18.928496485912,-11.5302951941811));
#87356=CARTESIAN_POINT('Ctrl Pts',(12.1079676069651,19.5944481184793,-11.9018501855925));
#87357=CARTESIAN_POINT('Ctrl Pts',(10.209624743653,20.6302930419102,-12.3957375602561));
#87358=CARTESIAN_POINT('Ctrl Pts',(9.35628286281192,21.0324554978147,-12.5583615922366));
#87359=CARTESIAN_POINT('Ctrl Pts',(8.47224530415855,21.3827280651035,-12.6858503806098));
#87360=CARTESIAN_POINT('',(23.3408711738295,21.3827280651035,-12.6858503806098));
#87361=CARTESIAN_POINT('',(0.,21.3827280651035,-12.6858503806098));
#87362=CARTESIAN_POINT('',(23.3408711739,30.6172719348965,-12.6858503806098));
#87363=CARTESIAN_POINT('Origin',(23.3408711739,26.,7.77156117237612E-15));
#87364=CARTESIAN_POINT('',(0.,30.6172719348965,-12.6858503806098));
#87365=CARTESIAN_POINT('Origin',(0.,34.3713153881227,-23.));
#87366=CARTESIAN_POINT('',(-23.341,26.,7.77156117237612E-15));
#87367=CARTESIAN_POINT('Origin',(0.,21.3827280651035,-12.6858503806098));
#87368=CARTESIAN_POINT('Origin',(0.,0.,-71.4344129058201));
#87369=CARTESIAN_POINT('',(23.341,26.,7.77156117237612E-15));
#87370=CARTESIAN_POINT('Origin',(0.,21.3827280651035,-12.6858503806098));
#87371=CARTESIAN_POINT('',(-23.341,26.,7.77156117237612E-15));
#87372=CARTESIAN_POINT('Origin',(0.,0.,-71.4344129058201));
#87373=CARTESIAN_POINT('Origin',(-23.341,26.,-17.8407788049984));
#87374=CARTESIAN_POINT('',(-23.341,22.,-12.8937969582276));
#87375=CARTESIAN_POINT('Origin',(-23.341,26.,7.77156117237612E-15));
#87376=CARTESIAN_POINT('Origin',(-23.3408711739,26.,7.77156117237612E-15));
#87377=CARTESIAN_POINT('Origin',(0.,34.3713153881227,-23.));
#87378=CARTESIAN_POINT('',(23.341,26.,7.77156117237612E-15));
#87379=CARTESIAN_POINT('Origin',(23.341,26.,-17.8407788049984));
#87380=CARTESIAN_POINT('Origin',(23.3408711739,26.,6.66133814775094E-15));
#87381=CARTESIAN_POINT('Origin',(-23.3408711739,26.,8.88178419700125E-15));
#87382=CARTESIAN_POINT('',(-23.3408711739,15.5,6.4856820332714E-15));
#87383=CARTESIAN_POINT('Origin',(-23.3408711739,26.,7.77156117237612E-15));
#87384=CARTESIAN_POINT('Origin',(-30.,51.,-23.));
#87385=CARTESIAN_POINT('',(-30.,-29.,-28.));
#87386=CARTESIAN_POINT('Origin',(0.,26.,7.77156117237612E-15));
#87387=CARTESIAN_POINT('',(-12.6392246597645,15.5,9.07151189591777E-15));
#87388=CARTESIAN_POINT('',(0.,15.5,6.4856820332714E-15));
#87389=CARTESIAN_POINT('',(0.,20.,-8.61684396980704));
#87390=CARTESIAN_POINT('Ctrl Pts',(-12.6392246597645,15.5,8.04911692853238E-15));
#87391=CARTESIAN_POINT('Ctrl Pts',(-12.6392246597645,15.5,-0.770455991080875));
#87392=CARTESIAN_POINT('Ctrl Pts',(-12.5292156787668,15.5917627320068,-1.59562994116201));
#87393=CARTESIAN_POINT('Ctrl Pts',(-12.0712736606586,15.9489399276083,-3.13904558498715));
#87394=CARTESIAN_POINT('Ctrl Pts',(-11.721971300226,16.2122340102582,-3.85737065648558));
#87395=CARTESIAN_POINT('Ctrl Pts',(-10.7496243003215,16.8795515666301,-5.2831275200831));
#87396=CARTESIAN_POINT('Ctrl Pts',(-10.0374064060355,17.3236709304054,-5.95380333582132));
#87397=CARTESIAN_POINT('Ctrl Pts',(-8.39213189202835,18.1777673238428,-7.03840434115244));
#87398=CARTESIAN_POINT('Ctrl Pts',(-7.45822274458716,18.5875681292269,-7.45117458755254));
#87399=CARTESIAN_POINT('Ctrl Pts',(-5.4523017781929,19.2716230475986,-8.07420868943815));
#87400=CARTESIAN_POINT('Ctrl Pts',(-4.37926194389239,19.546103021309,-8.28545463335066));
#87401=CARTESIAN_POINT('Ctrl Pts',(-2.19300975565939,19.91026838696,-8.55667651899198));
#87402=CARTESIAN_POINT('Ctrl Pts',(-1.07982886357284,20.,-8.61684396980704));
#87403=CARTESIAN_POINT('Ctrl Pts',(-2.77555756156289E-16,20.,-8.61684396980704));
#87404=CARTESIAN_POINT('',(12.6392246597645,15.5,7.33678841994096E-15));
#87405=CARTESIAN_POINT('Ctrl Pts',(0.,20.,-8.61684396980704));
#87406=CARTESIAN_POINT('Ctrl Pts',(1.07982886357284,20.,-8.61684396980704));
#87407=CARTESIAN_POINT('Ctrl Pts',(2.19300975565939,19.91026838696,-8.55667651899198));
#87408=CARTESIAN_POINT('Ctrl Pts',(4.37926194389239,19.546103021309,-8.28545463335066));
#87409=CARTESIAN_POINT('Ctrl Pts',(5.4523017781929,19.2716230475986,-8.07420868943815));
#87410=CARTESIAN_POINT('Ctrl Pts',(7.45822274458716,18.5875681292269,-7.45117458755254));
#87411=CARTESIAN_POINT('Ctrl Pts',(8.39213189202836,18.1777673238428,-7.03840434115244));
#87412=CARTESIAN_POINT('Ctrl Pts',(10.0374064060355,17.3236709304054,-5.95380333582132));
#87413=CARTESIAN_POINT('Ctrl Pts',(10.7496243003215,16.8795515666301,-5.2831275200831));
#87414=CARTESIAN_POINT('Ctrl Pts',(11.721971300226,16.2122340102582,-3.85737065648558));
#87415=CARTESIAN_POINT('Ctrl Pts',(12.0712736606586,15.9489399276083,-3.13904558498714));
#87416=CARTESIAN_POINT('Ctrl Pts',(12.5292156787668,15.5917627320068,-1.59562994116201));
#87417=CARTESIAN_POINT('Ctrl Pts',(12.6392246597645,15.5,-0.770455991080874));
#87418=CARTESIAN_POINT('Ctrl Pts',(12.6392246597645,15.5,8.32667268468867E-15));
#87419=CARTESIAN_POINT('',(23.3408711739,15.5,6.4856820332714E-15));
#87420=CARTESIAN_POINT('',(0.,15.5,6.4856820332714E-15));
#87421=CARTESIAN_POINT('Origin',(23.3408711739,26.,7.77156117237612E-15));
#87422=CARTESIAN_POINT('Ctrl Pts',(12.6392246597645,15.5,8.32667268468867E-15));
#87423=CARTESIAN_POINT('Ctrl Pts',(12.6392246597645,15.5,0.77045599108089));
#87424=CARTESIAN_POINT('Ctrl Pts',(12.5292156787668,15.5917627320068,1.59562994116203));
#87425=CARTESIAN_POINT('Ctrl Pts',(12.0712736606586,15.9489399276083,3.13904558498716));
#87426=CARTESIAN_POINT('Ctrl Pts',(11.721971300226,16.2122340102582,3.8573706564856));
#87427=CARTESIAN_POINT('Ctrl Pts',(10.7496243003215,16.8795515666301,5.28312752008312));
#87428=CARTESIAN_POINT('Ctrl Pts',(10.0374064060355,17.3236709304054,5.95380333582134));
#87429=CARTESIAN_POINT('Ctrl Pts',(8.39213189202835,18.1777673238429,7.03840434115246));
#87430=CARTESIAN_POINT('Ctrl Pts',(7.45822274458715,18.5875681292269,7.45117458755255));
#87431=CARTESIAN_POINT('Ctrl Pts',(5.4523017781929,19.2716230475986,8.07420868943816));
#87432=CARTESIAN_POINT('Ctrl Pts',(4.37926194389238,19.546103021309,8.28545463335068));
#87433=CARTESIAN_POINT('Ctrl Pts',(2.19300975565938,19.91026838696,8.556676518992));
#87434=CARTESIAN_POINT('Ctrl Pts',(1.07982886357284,20.,8.61684396980705));
#87435=CARTESIAN_POINT('Ctrl Pts',(0.,20.,8.61684396980705));
#87436=CARTESIAN_POINT('Ctrl Pts',(-1.07982886357284,20.,8.61684396980705));
#87437=CARTESIAN_POINT('Ctrl Pts',(-2.19300975565939,19.91026838696,8.556676518992));
#87438=CARTESIAN_POINT('Ctrl Pts',(-4.37926194389239,19.546103021309,8.28545463335068));
#87439=CARTESIAN_POINT('Ctrl Pts',(-5.4523017781929,19.2716230475986,8.07420868943816));
#87440=CARTESIAN_POINT('Ctrl Pts',(-7.45822274458715,18.5875681292269,7.45117458755255));
#87441=CARTESIAN_POINT('Ctrl Pts',(-8.39213189202835,18.1777673238429,7.03840434115246));
#87442=CARTESIAN_POINT('Ctrl Pts',(-10.0374064060354,17.3236709304054,5.95380333582134));
#87443=CARTESIAN_POINT('Ctrl Pts',(-10.7496243003215,16.8795515666301,5.28312752008312));
#87444=CARTESIAN_POINT('Ctrl Pts',(-11.721971300226,16.2122340102582,3.8573706564856));
#87445=CARTESIAN_POINT('Ctrl Pts',(-12.0712736606586,15.9489399276083,3.13904558498717));
#87446=CARTESIAN_POINT('Ctrl Pts',(-12.5292156787668,15.5917627320068,1.59562994116203));
#87447=CARTESIAN_POINT('Ctrl Pts',(-12.6392246597645,15.5,0.770455991080891));
#87448=CARTESIAN_POINT('Ctrl Pts',(-12.6392246597645,15.5,7.7715611723761E-15));
#87449=CARTESIAN_POINT('Origin',(0.,11.,-27.));
#87450=CARTESIAN_POINT('',(-20.,-2.44929359829471E-15,-27.));
#87451=CARTESIAN_POINT('Origin',(0.,0.,-27.));
#87452=CARTESIAN_POINT('Origin',(0.,0.,0.));
#87453=CARTESIAN_POINT('',(-20.,-2.44929359829471E-15,27.0000004769));
#87454=CARTESIAN_POINT('',(-20.,-2.44929359829471E-15,0.));
#87455=CARTESIAN_POINT('Origin',(0.,0.,27.0000004769));
#87456=CARTESIAN_POINT('Origin',(0.,0.,27.0000004769));
#87457=CARTESIAN_POINT('',(-23.,2.81668763803891E-15,27.0000004769));
#87458=CARTESIAN_POINT('Origin',(0.,0.,27.0000004769));
#87459=CARTESIAN_POINT('Origin',(0.,0.,0.));
#87460=CARTESIAN_POINT('',(-23.,-2.81668763803891E-15,0.));
#87461=CARTESIAN_POINT('Origin',(23.3408711739,26.,8.88178419700125E-15));
#87462=CARTESIAN_POINT('Origin',(0.,11.,-28.));
#88468=UNCERTAINTY_MEASURE_WITH_UNIT(LENGTH_MEASURE(0.01),#88484,
'DISTANCE_ACCURACY_VALUE',
'Maximum model space distance between geometric entities at asserted c
onnectivities');
#88472=UNCERTAINTY_MEASURE_WITH_UNIT(LENGTH_MEASURE(0.01),#88484,
'DISTANCE_ACCURACY_VALUE',
'Maximum model space distance between geometric entities at asserted c
onnectivities');
#88479=(
GEOMETRIC_REPRESENTATION_CONTEXT(3)
GLOBAL_UNCERTAINTY_ASSIGNED_CONTEXT((#88468))
GLOBAL_UNIT_ASSIGNED_CONTEXT((#88484,#88486,#88487))
REPRESENTATION_CONTEXT('','3D')
);
#88483=(
GEOMETRIC_REPRESENTATION_CONTEXT(3)
GLOBAL_UNCERTAINTY_ASSIGNED_CONTEXT((#88472))
GLOBAL_UNIT_ASSIGNED_CONTEXT((#88484,#88486,#88487))
REPRESENTATION_CONTEXT('','3D')
);
#88484=(
LENGTH_UNIT()
NAMED_UNIT(*)
SI_UNIT(.MILLI.,.METRE.)
);
#88486=(
NAMED_UNIT(*)
PLANE_ANGLE_UNIT()
SI_UNIT($,.RADIAN.)
);
#88487=(
NAMED_UNIT(*)
SI_UNIT($,.STERADIAN.)
SOLID_ANGLE_UNIT()
);
#88494=SHAPE_DEFINITION_REPRESENTATION(#88504,#88525);
#88504=PRODUCT_DEFINITION_SHAPE('',$,#88536);
#88525=SHAPE_REPRESENTATION('',(#13876),#88479);
#88529=PRODUCT_DEFINITION_CONTEXT('part definition',#88561,'design');
#88536=PRODUCT_DEFINITION('Housing','Housing',#88546,#88529);
#88546=PRODUCT_DEFINITION_FORMATION('',$,#88569);
#88561=APPLICATION_CONTEXT(
'Core Data for Automotive Mechanical Design Process');
#88562=PRODUCT_CONTEXT('part definition',#88561,'mechanical');
#88569=PRODUCT('Housing','Housing',$,(#88562));
#88574=PRESENTATION_STYLE_ASSIGNMENT((#88576));
#88576=SURFACE_STYLE_USAGE(.BOTH.,#88578);
#88578=SURFACE_SIDE_STYLE('',(#88580));
#88580=SURFACE_STYLE_FILL_AREA(#88582);
#88582=FILL_AREA_STYLE('Opaque(160,160,160)',(#88584));
#88584=FILL_AREA_STYLE_COLOUR('Opaque(160,160,160)',#88586);
#88586=COLOUR_RGB('Opaque(160,160,160)', 0.66274510, 0.83137255, 0.94901961);
ENDSEC;
END-ISO-10303-21;
